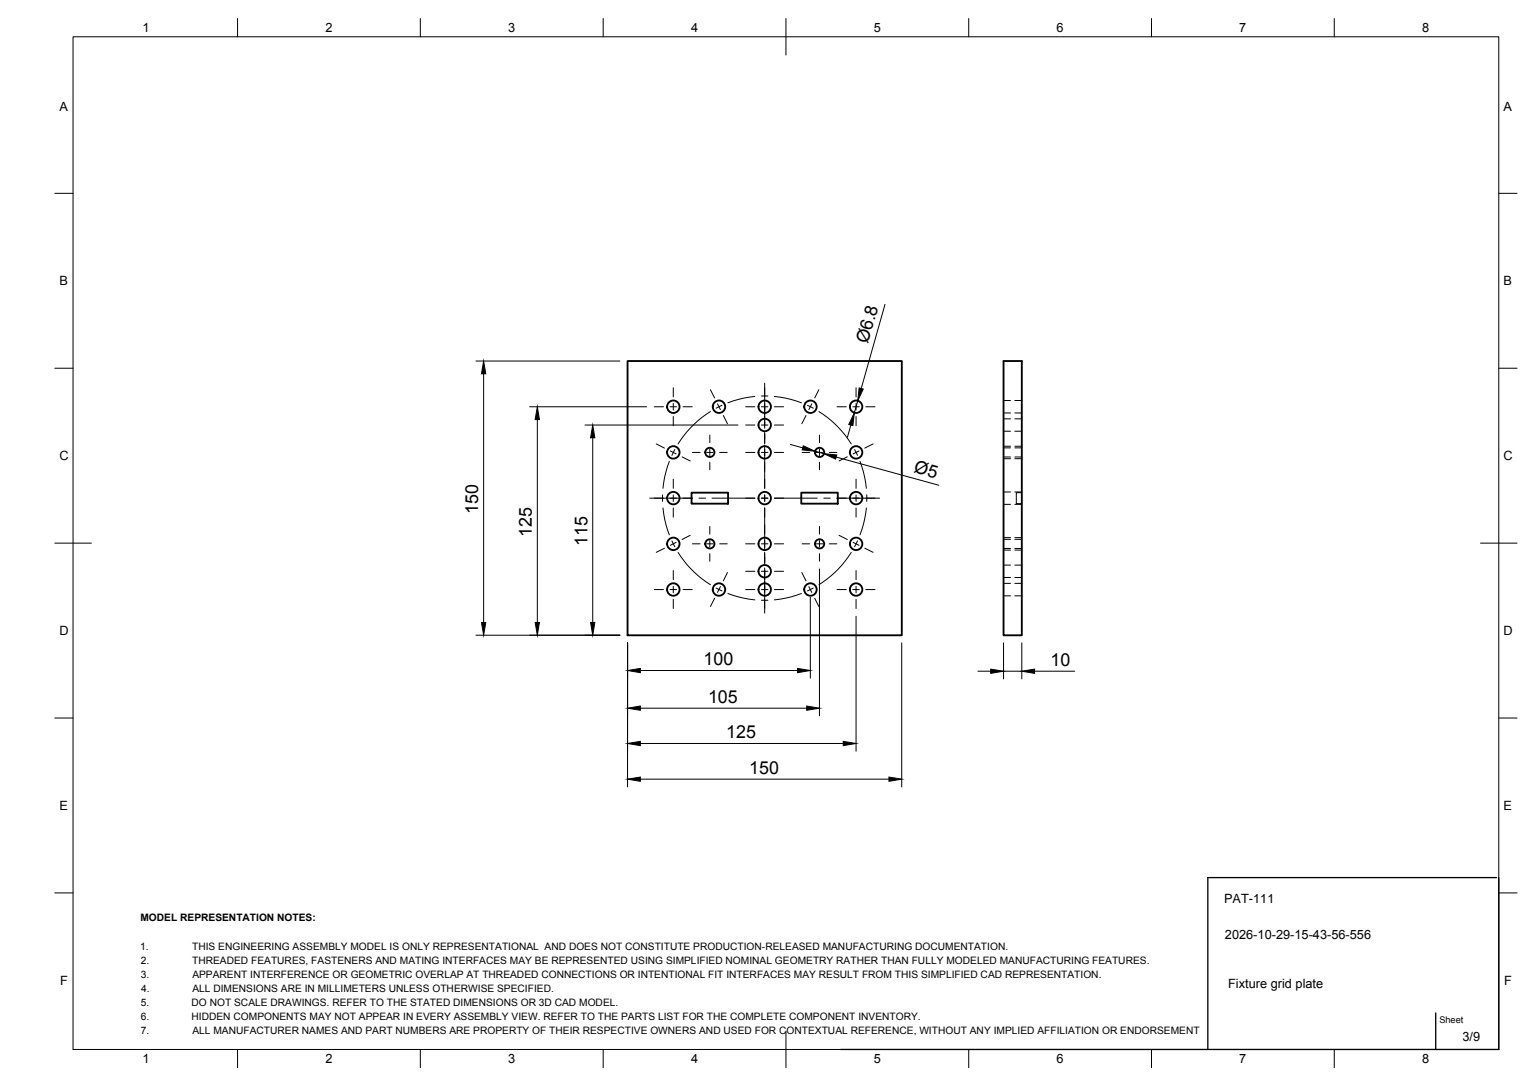
ISO-10303-21;
HEADER;
/* Generated by software containing ST-Developer
 * from STEP Tools, Inc. (www.steptools.com) 
 */

FILE_DESCRIPTION(
/* description */ ('Grid plate located blocks and clamp'),
/* implementation_level */ '2;1');

FILE_NAME(
/* name */ 'Fixture grid plate.step',
/* time_stamp */ '2026-10-29T15:43:47-07:00',
/* author */ (''),
/* organization */ (''),
/* preprocessor_version */ 'ST-DEVELOPER v20.2',
/* originating_system */ 'Autodesk Translation Framework v15.17.0.0',
/* authorisation */ '');

FILE_SCHEMA (('AUTOMOTIVE_DESIGN { 1 0 10303 214 3 1 1 }'));
ENDSEC;

DATA;
#10=MECHANICAL_DESIGN_GEOMETRIC_PRESENTATION_REPRESENTATION('',(#166),#5702);
#142=SHAPE_REPRESENTATION_RELATIONSHIP('SRR','None',#5760,#154);
#154=ADVANCED_BREP_SHAPE_REPRESENTATION('',(#180),#5690);
#166=STYLED_ITEM('',(#5911),#180);
#180=MANIFOLD_SOLID_BREP('Body1',#3261);
#192=FACE_BOUND('',#680,.T.);
#193=FACE_BOUND('',#681,.T.);
#194=FACE_BOUND('',#682,.T.);
#195=FACE_BOUND('',#683,.T.);
#196=FACE_BOUND('',#684,.T.);
#197=FACE_BOUND('',#685,.T.);
#198=FACE_BOUND('',#686,.T.);
#199=FACE_BOUND('',#687,.T.);
#200=FACE_BOUND('',#688,.T.);
#201=FACE_BOUND('',#689,.T.);
#202=FACE_BOUND('',#690,.T.);
#203=FACE_BOUND('',#691,.T.);
#204=FACE_BOUND('',#692,.T.);
#205=FACE_BOUND('',#693,.T.);
#206=FACE_BOUND('',#694,.T.);
#207=FACE_BOUND('',#695,.T.);
#208=FACE_BOUND('',#696,.T.);
#209=FACE_BOUND('',#697,.T.);
#210=FACE_BOUND('',#698,.T.);
#211=FACE_BOUND('',#699,.T.);
#212=FACE_BOUND('',#700,.T.);
#213=FACE_BOUND('',#701,.T.);
#214=FACE_BOUND('',#702,.T.);
#215=FACE_BOUND('',#703,.T.);
#216=FACE_BOUND('',#704,.T.);
#217=FACE_BOUND('',#705,.T.);
#218=FACE_BOUND('',#706,.T.);
#219=FACE_BOUND('',#708,.T.);
#220=FACE_BOUND('',#709,.T.);
#221=FACE_BOUND('',#710,.T.);
#222=FACE_BOUND('',#711,.T.);
#223=FACE_BOUND('',#712,.T.);
#224=FACE_BOUND('',#713,.T.);
#225=FACE_BOUND('',#714,.T.);
#226=FACE_BOUND('',#715,.T.);
#227=FACE_BOUND('',#716,.T.);
#228=FACE_BOUND('',#717,.T.);
#229=FACE_BOUND('',#718,.T.);
#230=FACE_BOUND('',#719,.T.);
#231=FACE_BOUND('',#720,.T.);
#232=FACE_BOUND('',#721,.T.);
#233=FACE_BOUND('',#722,.T.);
#234=FACE_BOUND('',#723,.T.);
#235=FACE_BOUND('',#724,.T.);
#236=FACE_BOUND('',#725,.T.);
#237=FACE_BOUND('',#726,.T.);
#238=FACE_BOUND('',#727,.T.);
#239=FACE_BOUND('',#728,.T.);
#240=FACE_BOUND('',#729,.T.);
#241=FACE_BOUND('',#730,.T.);
#242=FACE_BOUND('',#731,.T.);
#243=FACE_BOUND('',#732,.T.);
#268=CIRCLE('',#3423,0.25);
#269=CIRCLE('',#3424,0.25);
#270=CIRCLE('',#3426,0.25);
#271=CIRCLE('',#3427,0.25);
#272=CIRCLE('',#3429,0.25);
#273=CIRCLE('',#3430,0.25);
#274=CIRCLE('',#3432,0.25);
#275=CIRCLE('',#3433,0.25);
#276=CIRCLE('',#3435,0.34);
#277=CIRCLE('',#3436,0.34);
#278=CIRCLE('',#3438,0.34);
#279=CIRCLE('',#3439,0.34);
#280=CIRCLE('',#3441,0.34);
#281=CIRCLE('',#3442,0.34);
#282=CIRCLE('',#3444,0.34);
#283=CIRCLE('',#3445,0.34);
#284=CIRCLE('',#3447,0.34);
#285=CIRCLE('',#3448,0.34);
#286=CIRCLE('',#3450,0.34);
#287=CIRCLE('',#3451,0.34);
#288=CIRCLE('',#3453,0.34);
#289=CIRCLE('',#3454,0.34);
#290=CIRCLE('',#3456,0.34);
#291=CIRCLE('',#3457,0.34);
#292=CIRCLE('',#3459,0.34);
#293=CIRCLE('',#3460,0.34);
#294=CIRCLE('',#3462,0.34);
#295=CIRCLE('',#3463,0.34);
#296=CIRCLE('',#3465,0.34);
#297=CIRCLE('',#3466,0.34);
#298=CIRCLE('',#3468,0.34);
#299=CIRCLE('',#3469,0.34);
#300=CIRCLE('',#3471,0.34);
#301=CIRCLE('',#3472,0.34);
#302=CIRCLE('',#3474,0.34);
#303=CIRCLE('',#3475,0.34);
#304=CIRCLE('',#3477,0.34);
#305=CIRCLE('',#3478,0.34);
#306=CIRCLE('',#3480,0.34);
#307=CIRCLE('',#3481,0.34);
#308=CIRCLE('',#3483,0.34);
#309=CIRCLE('',#3484,0.34);
#310=CIRCLE('',#3486,0.34);
#311=CIRCLE('',#3487,0.34);
#312=CIRCLE('',#3489,0.34);
#313=CIRCLE('',#3490,0.34);
#314=CIRCLE('',#3492,0.34);
#315=CIRCLE('',#3493,0.34);
#316=CIRCLE('',#3495,0.34);
#317=CIRCLE('',#3496,0.34);
#397=CYLINDRICAL_SURFACE('',#3422,0.25);
#398=CYLINDRICAL_SURFACE('',#3425,0.25);
#399=CYLINDRICAL_SURFACE('',#3428,0.25);
#400=CYLINDRICAL_SURFACE('',#3431,0.25);
#401=CYLINDRICAL_SURFACE('',#3434,0.34);
#402=CYLINDRICAL_SURFACE('',#3437,0.34);
#403=CYLINDRICAL_SURFACE('',#3440,0.34);
#404=CYLINDRICAL_SURFACE('',#3443,0.34);
#405=CYLINDRICAL_SURFACE('',#3446,0.34);
#406=CYLINDRICAL_SURFACE('',#3449,0.34);
#407=CYLINDRICAL_SURFACE('',#3452,0.34);
#408=CYLINDRICAL_SURFACE('',#3455,0.34);
#409=CYLINDRICAL_SURFACE('',#3458,0.34);
#410=CYLINDRICAL_SURFACE('',#3461,0.34);
#411=CYLINDRICAL_SURFACE('',#3464,0.34);
#412=CYLINDRICAL_SURFACE('',#3467,0.34);
#413=CYLINDRICAL_SURFACE('',#3470,0.34);
#414=CYLINDRICAL_SURFACE('',#3473,0.34);
#415=CYLINDRICAL_SURFACE('',#3476,0.34);
#416=CYLINDRICAL_SURFACE('',#3479,0.34);
#417=CYLINDRICAL_SURFACE('',#3482,0.34);
#418=CYLINDRICAL_SURFACE('',#3485,0.34);
#419=CYLINDRICAL_SURFACE('',#3488,0.34);
#420=CYLINDRICAL_SURFACE('',#3491,0.34);
#421=CYLINDRICAL_SURFACE('',#3494,0.34);
#457=FACE_OUTER_BOUND('',#640,.T.);
#458=FACE_OUTER_BOUND('',#641,.T.);
#459=FACE_OUTER_BOUND('',#642,.T.);
#460=FACE_OUTER_BOUND('',#643,.T.);
#461=FACE_OUTER_BOUND('',#644,.T.);
#462=FACE_OUTER_BOUND('',#645,.T.);
#463=FACE_OUTER_BOUND('',#646,.T.);
#464=FACE_OUTER_BOUND('',#647,.T.);
#465=FACE_OUTER_BOUND('',#648,.T.);
#466=FACE_OUTER_BOUND('',#649,.T.);
#467=FACE_OUTER_BOUND('',#650,.T.);
#468=FACE_OUTER_BOUND('',#651,.T.);
#469=FACE_OUTER_BOUND('',#652,.T.);
#470=FACE_OUTER_BOUND('',#653,.T.);
#471=FACE_OUTER_BOUND('',#654,.T.);
#472=FACE_OUTER_BOUND('',#655,.T.);
#473=FACE_OUTER_BOUND('',#656,.T.);
#474=FACE_OUTER_BOUND('',#657,.T.);
#475=FACE_OUTER_BOUND('',#658,.T.);
#476=FACE_OUTER_BOUND('',#659,.T.);
#477=FACE_OUTER_BOUND('',#660,.T.);
#478=FACE_OUTER_BOUND('',#661,.T.);
#479=FACE_OUTER_BOUND('',#662,.T.);
#480=FACE_OUTER_BOUND('',#663,.T.);
#481=FACE_OUTER_BOUND('',#664,.T.);
#482=FACE_OUTER_BOUND('',#665,.T.);
#483=FACE_OUTER_BOUND('',#666,.T.);
#484=FACE_OUTER_BOUND('',#667,.T.);
#485=FACE_OUTER_BOUND('',#668,.T.);
#486=FACE_OUTER_BOUND('',#669,.T.);
#487=FACE_OUTER_BOUND('',#670,.T.);
#488=FACE_OUTER_BOUND('',#671,.T.);
#489=FACE_OUTER_BOUND('',#672,.T.);
#490=FACE_OUTER_BOUND('',#673,.T.);
#491=FACE_OUTER_BOUND('',#674,.T.);
#492=FACE_OUTER_BOUND('',#675,.T.);
#493=FACE_OUTER_BOUND('',#676,.T.);
#494=FACE_OUTER_BOUND('',#677,.T.);
#495=FACE_OUTER_BOUND('',#678,.T.);
#496=FACE_OUTER_BOUND('',#679,.T.);
#497=FACE_OUTER_BOUND('',#707,.T.);
#640=EDGE_LOOP('',(#2132,#2133,#2134,#2135));
#641=EDGE_LOOP('',(#2136,#2137,#2138,#2139));
#642=EDGE_LOOP('',(#2140,#2141,#2142,#2143));
#643=EDGE_LOOP('',(#2144,#2145,#2146,#2147));
#644=EDGE_LOOP('',(#2148,#2149,#2150,#2151));
#645=EDGE_LOOP('',(#2152,#2153,#2154,#2155));
#646=EDGE_LOOP('',(#2156,#2157,#2158,#2159));
#647=EDGE_LOOP('',(#2160,#2161,#2162,#2163));
#648=EDGE_LOOP('',(#2164,#2165,#2166,#2167));
#649=EDGE_LOOP('',(#2168,#2169,#2170,#2171));
#650=EDGE_LOOP('',(#2172,#2173,#2174,#2175));
#651=EDGE_LOOP('',(#2176,#2177,#2178,#2179));
#652=EDGE_LOOP('',(#2180,#2181,#2182,#2183));
#653=EDGE_LOOP('',(#2184,#2185,#2186,#2187));
#654=EDGE_LOOP('',(#2188,#2189,#2190,#2191));
#655=EDGE_LOOP('',(#2192,#2193,#2194,#2195));
#656=EDGE_LOOP('',(#2196,#2197,#2198,#2199));
#657=EDGE_LOOP('',(#2200,#2201,#2202,#2203));
#658=EDGE_LOOP('',(#2204,#2205,#2206,#2207));
#659=EDGE_LOOP('',(#2208,#2209,#2210,#2211));
#660=EDGE_LOOP('',(#2212,#2213,#2214,#2215));
#661=EDGE_LOOP('',(#2216,#2217,#2218,#2219));
#662=EDGE_LOOP('',(#2220,#2221,#2222,#2223));
#663=EDGE_LOOP('',(#2224,#2225,#2226,#2227));
#664=EDGE_LOOP('',(#2228,#2229,#2230,#2231));
#665=EDGE_LOOP('',(#2232,#2233,#2234,#2235));
#666=EDGE_LOOP('',(#2236,#2237,#2238,#2239));
#667=EDGE_LOOP('',(#2240,#2241,#2242,#2243));
#668=EDGE_LOOP('',(#2244,#2245,#2246,#2247));
#669=EDGE_LOOP('',(#2248,#2249,#2250,#2251));
#670=EDGE_LOOP('',(#2252,#2253,#2254,#2255));
#671=EDGE_LOOP('',(#2256,#2257,#2258,#2259));
#672=EDGE_LOOP('',(#2260,#2261,#2262,#2263));
#673=EDGE_LOOP('',(#2264,#2265,#2266,#2267));
#674=EDGE_LOOP('',(#2268,#2269,#2270,#2271));
#675=EDGE_LOOP('',(#2272,#2273,#2274,#2275));
#676=EDGE_LOOP('',(#2276,#2277,#2278,#2279));
#677=EDGE_LOOP('',(#2280,#2281,#2282,#2283));
#678=EDGE_LOOP('',(#2284,#2285,#2286,#2287));
#679=EDGE_LOOP('',(#2288,#2289,#2290,#2291));
#680=EDGE_LOOP('',(#2292,#2293,#2294,#2295));
#681=EDGE_LOOP('',(#2296));
#682=EDGE_LOOP('',(#2297));
#683=EDGE_LOOP('',(#2298));
#684=EDGE_LOOP('',(#2299));
#685=EDGE_LOOP('',(#2300));
#686=EDGE_LOOP('',(#2301));
#687=EDGE_LOOP('',(#2302));
#688=EDGE_LOOP('',(#2303));
#689=EDGE_LOOP('',(#2304));
#690=EDGE_LOOP('',(#2305));
#691=EDGE_LOOP('',(#2306));
#692=EDGE_LOOP('',(#2307));
#693=EDGE_LOOP('',(#2308));
#694=EDGE_LOOP('',(#2309));
#695=EDGE_LOOP('',(#2310));
#696=EDGE_LOOP('',(#2311));
#697=EDGE_LOOP('',(#2312));
#698=EDGE_LOOP('',(#2313));
#699=EDGE_LOOP('',(#2314));
#700=EDGE_LOOP('',(#2315));
#701=EDGE_LOOP('',(#2316));
#702=EDGE_LOOP('',(#2317));
#703=EDGE_LOOP('',(#2318));
#704=EDGE_LOOP('',(#2319));
#705=EDGE_LOOP('',(#2320));
#706=EDGE_LOOP('',(#2321,#2322,#2323,#2324));
#707=EDGE_LOOP('',(#2325,#2326,#2327,#2328));
#708=EDGE_LOOP('',(#2329));
#709=EDGE_LOOP('',(#2330));
#710=EDGE_LOOP('',(#2331));
#711=EDGE_LOOP('',(#2332));
#712=EDGE_LOOP('',(#2333));
#713=EDGE_LOOP('',(#2334));
#714=EDGE_LOOP('',(#2335));
#715=EDGE_LOOP('',(#2336));
#716=EDGE_LOOP('',(#2337));
#717=EDGE_LOOP('',(#2338));
#718=EDGE_LOOP('',(#2339));
#719=EDGE_LOOP('',(#2340));
#720=EDGE_LOOP('',(#2341));
#721=EDGE_LOOP('',(#2342));
#722=EDGE_LOOP('',(#2343));
#723=EDGE_LOOP('',(#2344));
#724=EDGE_LOOP('',(#2345));
#725=EDGE_LOOP('',(#2346));
#726=EDGE_LOOP('',(#2347));
#727=EDGE_LOOP('',(#2348));
#728=EDGE_LOOP('',(#2349));
#729=EDGE_LOOP('',(#2350));
#730=EDGE_LOOP('',(#2351));
#731=EDGE_LOOP('',(#2352));
#732=EDGE_LOOP('',(#2353));
#899=LINE('',#4747,#1172);
#900=LINE('',#4749,#1173);
#901=LINE('',#4751,#1174);
#902=LINE('',#4752,#1175);
#903=LINE('',#4755,#1176);
#904=LINE('',#4757,#1177);
#905=LINE('',#4758,#1178);
#906=LINE('',#4761,#1179);
#907=LINE('',#4763,#1180);
#908=LINE('',#4764,#1181);
#909=LINE('',#4766,#1182);
#910=LINE('',#4767,#1183);
#911=LINE('',#4772,#1184);
#912=LINE('',#4774,#1185);
#913=LINE('',#4776,#1186);
#914=LINE('',#4777,#1187);
#915=LINE('',#4780,#1188);
#916=LINE('',#4782,#1189);
#917=LINE('',#4783,#1190);
#918=LINE('',#4786,#1191);
#919=LINE('',#4788,#1192);
#920=LINE('',#4789,#1193);
#921=LINE('',#4791,#1194);
#922=LINE('',#4792,#1195);
#923=LINE('',#4798,#1196);
#924=LINE('',#4804,#1197);
#925=LINE('',#4810,#1198);
#926=LINE('',#4816,#1199);
#927=LINE('',#4822,#1200);
#928=LINE('',#4828,#1201);
#929=LINE('',#4834,#1202);
#930=LINE('',#4840,#1203);
#931=LINE('',#4846,#1204);
#932=LINE('',#4852,#1205);
#933=LINE('',#4858,#1206);
#934=LINE('',#4864,#1207);
#935=LINE('',#4870,#1208);
#936=LINE('',#4876,#1209);
#937=LINE('',#4882,#1210);
#938=LINE('',#4888,#1211);
#939=LINE('',#4894,#1212);
#940=LINE('',#4900,#1213);
#941=LINE('',#4906,#1214);
#942=LINE('',#4912,#1215);
#943=LINE('',#4918,#1216);
#944=LINE('',#4924,#1217);
#945=LINE('',#4930,#1218);
#946=LINE('',#4936,#1219);
#947=LINE('',#4942,#1220);
#948=LINE('',#4947,#1221);
#949=LINE('',#4949,#1222);
#950=LINE('',#4951,#1223);
#951=LINE('',#4952,#1224);
#952=LINE('',#4955,#1225);
#953=LINE('',#4957,#1226);
#954=LINE('',#4958,#1227);
#955=LINE('',#4961,#1228);
#956=LINE('',#4963,#1229);
#957=LINE('',#4964,#1230);
#958=LINE('',#4966,#1231);
#959=LINE('',#4967,#1232);
#1172=VECTOR('',#3769,1.);
#1173=VECTOR('',#3770,1.);
#1174=VECTOR('',#3771,1.);
#1175=VECTOR('',#3772,1.);
#1176=VECTOR('',#3775,1.);
#1177=VECTOR('',#3776,1.);
#1178=VECTOR('',#3777,1.);
#1179=VECTOR('',#3780,1.);
#1180=VECTOR('',#3781,1.);
#1181=VECTOR('',#3782,1.);
#1182=VECTOR('',#3785,1.);
#1183=VECTOR('',#3786,1.);
#1184=VECTOR('',#3791,1.);
#1185=VECTOR('',#3792,1.);
#1186=VECTOR('',#3793,1.);
#1187=VECTOR('',#3794,1.);
#1188=VECTOR('',#3797,1.);
#1189=VECTOR('',#3798,1.);
#1190=VECTOR('',#3799,1.);
#1191=VECTOR('',#3802,1.);
#1192=VECTOR('',#3803,1.);
#1193=VECTOR('',#3804,1.);
#1194=VECTOR('',#3807,1.);
#1195=VECTOR('',#3808,1.);
#1196=VECTOR('',#3815,0.25);
#1197=VECTOR('',#3822,0.25);
#1198=VECTOR('',#3829,0.25);
#1199=VECTOR('',#3836,0.25);
#1200=VECTOR('',#3843,0.34);
#1201=VECTOR('',#3850,0.34);
#1202=VECTOR('',#3857,0.34);
#1203=VECTOR('',#3864,0.34);
#1204=VECTOR('',#3871,0.34);
#1205=VECTOR('',#3878,0.34);
#1206=VECTOR('',#3885,0.34);
#1207=VECTOR('',#3892,0.34);
#1208=VECTOR('',#3899,0.34);
#1209=VECTOR('',#3906,0.34);
#1210=VECTOR('',#3913,0.34);
#1211=VECTOR('',#3920,0.34);
#1212=VECTOR('',#3927,0.34);
#1213=VECTOR('',#3934,0.34);
#1214=VECTOR('',#3941,0.34);
#1215=VECTOR('',#3948,0.34);
#1216=VECTOR('',#3955,0.34);
#1217=VECTOR('',#3962,0.34);
#1218=VECTOR('',#3969,0.34);
#1219=VECTOR('',#3976,0.34);
#1220=VECTOR('',#3983,0.34);
#1221=VECTOR('',#3988,1.);
#1222=VECTOR('',#3989,1.);
#1223=VECTOR('',#3990,1.);
#1224=VECTOR('',#3991,1.);
#1225=VECTOR('',#3994,1.);
#1226=VECTOR('',#3995,1.);
#1227=VECTOR('',#3996,1.);
#1228=VECTOR('',#3999,1.);
#1229=VECTOR('',#4000,1.);
#1230=VECTOR('',#4001,1.);
#1231=VECTOR('',#4004,1.);
#1232=VECTOR('',#4005,1.);
#1445=VERTEX_POINT('',#4745);
#1446=VERTEX_POINT('',#4746);
#1447=VERTEX_POINT('',#4748);
#1448=VERTEX_POINT('',#4750);
#1449=VERTEX_POINT('',#4754);
#1450=VERTEX_POINT('',#4756);
#1451=VERTEX_POINT('',#4760);
#1452=VERTEX_POINT('',#4762);
#1453=VERTEX_POINT('',#4770);
#1454=VERTEX_POINT('',#4771);
#1455=VERTEX_POINT('',#4773);
#1456=VERTEX_POINT('',#4775);
#1457=VERTEX_POINT('',#4779);
#1458=VERTEX_POINT('',#4781);
#1459=VERTEX_POINT('',#4785);
#1460=VERTEX_POINT('',#4787);
#1461=VERTEX_POINT('',#4795);
#1462=VERTEX_POINT('',#4797);
#1463=VERTEX_POINT('',#4801);
#1464=VERTEX_POINT('',#4803);
#1465=VERTEX_POINT('',#4807);
#1466=VERTEX_POINT('',#4809);
#1467=VERTEX_POINT('',#4813);
#1468=VERTEX_POINT('',#4815);
#1469=VERTEX_POINT('',#4819);
#1470=VERTEX_POINT('',#4821);
#1471=VERTEX_POINT('',#4825);
#1472=VERTEX_POINT('',#4827);
#1473=VERTEX_POINT('',#4831);
#1474=VERTEX_POINT('',#4833);
#1475=VERTEX_POINT('',#4837);
#1476=VERTEX_POINT('',#4839);
#1477=VERTEX_POINT('',#4843);
#1478=VERTEX_POINT('',#4845);
#1479=VERTEX_POINT('',#4849);
#1480=VERTEX_POINT('',#4851);
#1481=VERTEX_POINT('',#4855);
#1482=VERTEX_POINT('',#4857);
#1483=VERTEX_POINT('',#4861);
#1484=VERTEX_POINT('',#4863);
#1485=VERTEX_POINT('',#4867);
#1486=VERTEX_POINT('',#4869);
#1487=VERTEX_POINT('',#4873);
#1488=VERTEX_POINT('',#4875);
#1489=VERTEX_POINT('',#4879);
#1490=VERTEX_POINT('',#4881);
#1491=VERTEX_POINT('',#4885);
#1492=VERTEX_POINT('',#4887);
#1493=VERTEX_POINT('',#4891);
#1494=VERTEX_POINT('',#4893);
#1495=VERTEX_POINT('',#4897);
#1496=VERTEX_POINT('',#4899);
#1497=VERTEX_POINT('',#4903);
#1498=VERTEX_POINT('',#4905);
#1499=VERTEX_POINT('',#4909);
#1500=VERTEX_POINT('',#4911);
#1501=VERTEX_POINT('',#4915);
#1502=VERTEX_POINT('',#4917);
#1503=VERTEX_POINT('',#4921);
#1504=VERTEX_POINT('',#4923);
#1505=VERTEX_POINT('',#4927);
#1506=VERTEX_POINT('',#4929);
#1507=VERTEX_POINT('',#4933);
#1508=VERTEX_POINT('',#4935);
#1509=VERTEX_POINT('',#4939);
#1510=VERTEX_POINT('',#4941);
#1511=VERTEX_POINT('',#4945);
#1512=VERTEX_POINT('',#4946);
#1513=VERTEX_POINT('',#4948);
#1514=VERTEX_POINT('',#4950);
#1515=VERTEX_POINT('',#4954);
#1516=VERTEX_POINT('',#4956);
#1517=VERTEX_POINT('',#4960);
#1518=VERTEX_POINT('',#4962);
#1716=EDGE_CURVE('',#1445,#1446,#899,.T.);
#1717=EDGE_CURVE('',#1447,#1445,#900,.T.);
#1718=EDGE_CURVE('',#1448,#1447,#901,.T.);
#1719=EDGE_CURVE('',#1448,#1446,#902,.T.);
#1720=EDGE_CURVE('',#1446,#1449,#903,.T.);
#1721=EDGE_CURVE('',#1450,#1448,#904,.T.);
#1722=EDGE_CURVE('',#1450,#1449,#905,.T.);
#1723=EDGE_CURVE('',#1449,#1451,#906,.T.);
#1724=EDGE_CURVE('',#1452,#1450,#907,.T.);
#1725=EDGE_CURVE('',#1452,#1451,#908,.T.);
#1726=EDGE_CURVE('',#1451,#1445,#909,.T.);
#1727=EDGE_CURVE('',#1447,#1452,#910,.T.);
#1728=EDGE_CURVE('',#1453,#1454,#911,.T.);
#1729=EDGE_CURVE('',#1455,#1453,#912,.T.);
#1730=EDGE_CURVE('',#1456,#1455,#913,.T.);
#1731=EDGE_CURVE('',#1456,#1454,#914,.T.);
#1732=EDGE_CURVE('',#1454,#1457,#915,.T.);
#1733=EDGE_CURVE('',#1458,#1456,#916,.T.);
#1734=EDGE_CURVE('',#1458,#1457,#917,.T.);
#1735=EDGE_CURVE('',#1457,#1459,#918,.T.);
#1736=EDGE_CURVE('',#1460,#1458,#919,.T.);
#1737=EDGE_CURVE('',#1460,#1459,#920,.T.);
#1738=EDGE_CURVE('',#1459,#1453,#921,.T.);
#1739=EDGE_CURVE('',#1455,#1460,#922,.T.);
#1740=EDGE_CURVE('',#1461,#1461,#268,.T.);
#1741=EDGE_CURVE('',#1461,#1462,#923,.T.);
#1742=EDGE_CURVE('',#1462,#1462,#269,.T.);
#1743=EDGE_CURVE('',#1463,#1463,#270,.T.);
#1744=EDGE_CURVE('',#1463,#1464,#924,.T.);
#1745=EDGE_CURVE('',#1464,#1464,#271,.T.);
#1746=EDGE_CURVE('',#1465,#1465,#272,.T.);
#1747=EDGE_CURVE('',#1465,#1466,#925,.T.);
#1748=EDGE_CURVE('',#1466,#1466,#273,.T.);
#1749=EDGE_CURVE('',#1467,#1467,#274,.T.);
#1750=EDGE_CURVE('',#1467,#1468,#926,.T.);
#1751=EDGE_CURVE('',#1468,#1468,#275,.T.);
#1752=EDGE_CURVE('',#1469,#1469,#276,.T.);
#1753=EDGE_CURVE('',#1469,#1470,#927,.T.);
#1754=EDGE_CURVE('',#1470,#1470,#277,.T.);
#1755=EDGE_CURVE('',#1471,#1471,#278,.T.);
#1756=EDGE_CURVE('',#1471,#1472,#928,.T.);
#1757=EDGE_CURVE('',#1472,#1472,#279,.T.);
#1758=EDGE_CURVE('',#1473,#1473,#280,.T.);
#1759=EDGE_CURVE('',#1473,#1474,#929,.T.);
#1760=EDGE_CURVE('',#1474,#1474,#281,.T.);
#1761=EDGE_CURVE('',#1475,#1475,#282,.T.);
#1762=EDGE_CURVE('',#1475,#1476,#930,.T.);
#1763=EDGE_CURVE('',#1476,#1476,#283,.T.);
#1764=EDGE_CURVE('',#1477,#1477,#284,.T.);
#1765=EDGE_CURVE('',#1477,#1478,#931,.T.);
#1766=EDGE_CURVE('',#1478,#1478,#285,.T.);
#1767=EDGE_CURVE('',#1479,#1479,#286,.T.);
#1768=EDGE_CURVE('',#1479,#1480,#932,.T.);
#1769=EDGE_CURVE('',#1480,#1480,#287,.T.);
#1770=EDGE_CURVE('',#1481,#1481,#288,.T.);
#1771=EDGE_CURVE('',#1481,#1482,#933,.T.);
#1772=EDGE_CURVE('',#1482,#1482,#289,.T.);
#1773=EDGE_CURVE('',#1483,#1483,#290,.T.);
#1774=EDGE_CURVE('',#1483,#1484,#934,.T.);
#1775=EDGE_CURVE('',#1484,#1484,#291,.T.);
#1776=EDGE_CURVE('',#1485,#1485,#292,.T.);
#1777=EDGE_CURVE('',#1485,#1486,#935,.T.);
#1778=EDGE_CURVE('',#1486,#1486,#293,.T.);
#1779=EDGE_CURVE('',#1487,#1487,#294,.T.);
#1780=EDGE_CURVE('',#1487,#1488,#936,.T.);
#1781=EDGE_CURVE('',#1488,#1488,#295,.T.);
#1782=EDGE_CURVE('',#1489,#1489,#296,.T.);
#1783=EDGE_CURVE('',#1489,#1490,#937,.T.);
#1784=EDGE_CURVE('',#1490,#1490,#297,.T.);
#1785=EDGE_CURVE('',#1491,#1491,#298,.T.);
#1786=EDGE_CURVE('',#1491,#1492,#938,.T.);
#1787=EDGE_CURVE('',#1492,#1492,#299,.T.);
#1788=EDGE_CURVE('',#1493,#1493,#300,.T.);
#1789=EDGE_CURVE('',#1493,#1494,#939,.T.);
#1790=EDGE_CURVE('',#1494,#1494,#301,.T.);
#1791=EDGE_CURVE('',#1495,#1495,#302,.T.);
#1792=EDGE_CURVE('',#1495,#1496,#940,.T.);
#1793=EDGE_CURVE('',#1496,#1496,#303,.T.);
#1794=EDGE_CURVE('',#1497,#1497,#304,.T.);
#1795=EDGE_CURVE('',#1497,#1498,#941,.T.);
#1796=EDGE_CURVE('',#1498,#1498,#305,.T.);
#1797=EDGE_CURVE('',#1499,#1499,#306,.T.);
#1798=EDGE_CURVE('',#1499,#1500,#942,.T.);
#1799=EDGE_CURVE('',#1500,#1500,#307,.T.);
#1800=EDGE_CURVE('',#1501,#1501,#308,.T.);
#1801=EDGE_CURVE('',#1501,#1502,#943,.T.);
#1802=EDGE_CURVE('',#1502,#1502,#309,.T.);
#1803=EDGE_CURVE('',#1503,#1503,#310,.T.);
#1804=EDGE_CURVE('',#1503,#1504,#944,.T.);
#1805=EDGE_CURVE('',#1504,#1504,#311,.T.);
#1806=EDGE_CURVE('',#1505,#1505,#312,.T.);
#1807=EDGE_CURVE('',#1505,#1506,#945,.T.);
#1808=EDGE_CURVE('',#1506,#1506,#313,.T.);
#1809=EDGE_CURVE('',#1507,#1507,#314,.T.);
#1810=EDGE_CURVE('',#1507,#1508,#946,.T.);
#1811=EDGE_CURVE('',#1508,#1508,#315,.T.);
#1812=EDGE_CURVE('',#1509,#1509,#316,.T.);
#1813=EDGE_CURVE('',#1509,#1510,#947,.T.);
#1814=EDGE_CURVE('',#1510,#1510,#317,.T.);
#1815=EDGE_CURVE('',#1511,#1512,#948,.T.);
#1816=EDGE_CURVE('',#1512,#1513,#949,.T.);
#1817=EDGE_CURVE('',#1514,#1513,#950,.T.);
#1818=EDGE_CURVE('',#1511,#1514,#951,.T.);
#1819=EDGE_CURVE('',#1515,#1511,#952,.T.);
#1820=EDGE_CURVE('',#1516,#1514,#953,.T.);
#1821=EDGE_CURVE('',#1515,#1516,#954,.T.);
#1822=EDGE_CURVE('',#1517,#1515,#955,.T.);
#1823=EDGE_CURVE('',#1518,#1516,#956,.T.);
#1824=EDGE_CURVE('',#1517,#1518,#957,.T.);
#1825=EDGE_CURVE('',#1512,#1517,#958,.T.);
#1826=EDGE_CURVE('',#1513,#1518,#959,.T.);
#2132=ORIENTED_EDGE('',*,*,#1716,.F.);
#2133=ORIENTED_EDGE('',*,*,#1717,.F.);
#2134=ORIENTED_EDGE('',*,*,#1718,.F.);
#2135=ORIENTED_EDGE('',*,*,#1719,.T.);
#2136=ORIENTED_EDGE('',*,*,#1720,.F.);
#2137=ORIENTED_EDGE('',*,*,#1719,.F.);
#2138=ORIENTED_EDGE('',*,*,#1721,.F.);
#2139=ORIENTED_EDGE('',*,*,#1722,.T.);
#2140=ORIENTED_EDGE('',*,*,#1723,.F.);
#2141=ORIENTED_EDGE('',*,*,#1722,.F.);
#2142=ORIENTED_EDGE('',*,*,#1724,.F.);
#2143=ORIENTED_EDGE('',*,*,#1725,.T.);
#2144=ORIENTED_EDGE('',*,*,#1726,.F.);
#2145=ORIENTED_EDGE('',*,*,#1725,.F.);
#2146=ORIENTED_EDGE('',*,*,#1727,.F.);
#2147=ORIENTED_EDGE('',*,*,#1717,.T.);
#2148=ORIENTED_EDGE('',*,*,#1721,.T.);
#2149=ORIENTED_EDGE('',*,*,#1718,.T.);
#2150=ORIENTED_EDGE('',*,*,#1727,.T.);
#2151=ORIENTED_EDGE('',*,*,#1724,.T.);
#2152=ORIENTED_EDGE('',*,*,#1728,.F.);
#2153=ORIENTED_EDGE('',*,*,#1729,.F.);
#2154=ORIENTED_EDGE('',*,*,#1730,.F.);
#2155=ORIENTED_EDGE('',*,*,#1731,.T.);
#2156=ORIENTED_EDGE('',*,*,#1732,.F.);
#2157=ORIENTED_EDGE('',*,*,#1731,.F.);
#2158=ORIENTED_EDGE('',*,*,#1733,.F.);
#2159=ORIENTED_EDGE('',*,*,#1734,.T.);
#2160=ORIENTED_EDGE('',*,*,#1735,.F.);
#2161=ORIENTED_EDGE('',*,*,#1734,.F.);
#2162=ORIENTED_EDGE('',*,*,#1736,.F.);
#2163=ORIENTED_EDGE('',*,*,#1737,.T.);
#2164=ORIENTED_EDGE('',*,*,#1738,.F.);
#2165=ORIENTED_EDGE('',*,*,#1737,.F.);
#2166=ORIENTED_EDGE('',*,*,#1739,.F.);
#2167=ORIENTED_EDGE('',*,*,#1729,.T.);
#2168=ORIENTED_EDGE('',*,*,#1733,.T.);
#2169=ORIENTED_EDGE('',*,*,#1730,.T.);
#2170=ORIENTED_EDGE('',*,*,#1739,.T.);
#2171=ORIENTED_EDGE('',*,*,#1736,.T.);
#2172=ORIENTED_EDGE('',*,*,#1740,.F.);
#2173=ORIENTED_EDGE('',*,*,#1741,.T.);
#2174=ORIENTED_EDGE('',*,*,#1742,.F.);
#2175=ORIENTED_EDGE('',*,*,#1741,.F.);
#2176=ORIENTED_EDGE('',*,*,#1743,.F.);
#2177=ORIENTED_EDGE('',*,*,#1744,.T.);
#2178=ORIENTED_EDGE('',*,*,#1745,.F.);
#2179=ORIENTED_EDGE('',*,*,#1744,.F.);
#2180=ORIENTED_EDGE('',*,*,#1746,.F.);
#2181=ORIENTED_EDGE('',*,*,#1747,.T.);
#2182=ORIENTED_EDGE('',*,*,#1748,.F.);
#2183=ORIENTED_EDGE('',*,*,#1747,.F.);
#2184=ORIENTED_EDGE('',*,*,#1749,.F.);
#2185=ORIENTED_EDGE('',*,*,#1750,.T.);
#2186=ORIENTED_EDGE('',*,*,#1751,.F.);
#2187=ORIENTED_EDGE('',*,*,#1750,.F.);
#2188=ORIENTED_EDGE('',*,*,#1752,.F.);
#2189=ORIENTED_EDGE('',*,*,#1753,.T.);
#2190=ORIENTED_EDGE('',*,*,#1754,.F.);
#2191=ORIENTED_EDGE('',*,*,#1753,.F.);
#2192=ORIENTED_EDGE('',*,*,#1755,.F.);
#2193=ORIENTED_EDGE('',*,*,#1756,.T.);
#2194=ORIENTED_EDGE('',*,*,#1757,.F.);
#2195=ORIENTED_EDGE('',*,*,#1756,.F.);
#2196=ORIENTED_EDGE('',*,*,#1758,.F.);
#2197=ORIENTED_EDGE('',*,*,#1759,.T.);
#2198=ORIENTED_EDGE('',*,*,#1760,.F.);
#2199=ORIENTED_EDGE('',*,*,#1759,.F.);
#2200=ORIENTED_EDGE('',*,*,#1761,.F.);
#2201=ORIENTED_EDGE('',*,*,#1762,.T.);
#2202=ORIENTED_EDGE('',*,*,#1763,.F.);
#2203=ORIENTED_EDGE('',*,*,#1762,.F.);
#2204=ORIENTED_EDGE('',*,*,#1764,.F.);
#2205=ORIENTED_EDGE('',*,*,#1765,.T.);
#2206=ORIENTED_EDGE('',*,*,#1766,.F.);
#2207=ORIENTED_EDGE('',*,*,#1765,.F.);
#2208=ORIENTED_EDGE('',*,*,#1767,.F.);
#2209=ORIENTED_EDGE('',*,*,#1768,.T.);
#2210=ORIENTED_EDGE('',*,*,#1769,.F.);
#2211=ORIENTED_EDGE('',*,*,#1768,.F.);
#2212=ORIENTED_EDGE('',*,*,#1770,.F.);
#2213=ORIENTED_EDGE('',*,*,#1771,.T.);
#2214=ORIENTED_EDGE('',*,*,#1772,.F.);
#2215=ORIENTED_EDGE('',*,*,#1771,.F.);
#2216=ORIENTED_EDGE('',*,*,#1773,.F.);
#2217=ORIENTED_EDGE('',*,*,#1774,.T.);
#2218=ORIENTED_EDGE('',*,*,#1775,.F.);
#2219=ORIENTED_EDGE('',*,*,#1774,.F.);
#2220=ORIENTED_EDGE('',*,*,#1776,.F.);
#2221=ORIENTED_EDGE('',*,*,#1777,.T.);
#2222=ORIENTED_EDGE('',*,*,#1778,.F.);
#2223=ORIENTED_EDGE('',*,*,#1777,.F.);
#2224=ORIENTED_EDGE('',*,*,#1779,.F.);
#2225=ORIENTED_EDGE('',*,*,#1780,.T.);
#2226=ORIENTED_EDGE('',*,*,#1781,.F.);
#2227=ORIENTED_EDGE('',*,*,#1780,.F.);
#2228=ORIENTED_EDGE('',*,*,#1782,.F.);
#2229=ORIENTED_EDGE('',*,*,#1783,.T.);
#2230=ORIENTED_EDGE('',*,*,#1784,.F.);
#2231=ORIENTED_EDGE('',*,*,#1783,.F.);
#2232=ORIENTED_EDGE('',*,*,#1785,.F.);
#2233=ORIENTED_EDGE('',*,*,#1786,.T.);
#2234=ORIENTED_EDGE('',*,*,#1787,.F.);
#2235=ORIENTED_EDGE('',*,*,#1786,.F.);
#2236=ORIENTED_EDGE('',*,*,#1788,.F.);
#2237=ORIENTED_EDGE('',*,*,#1789,.T.);
#2238=ORIENTED_EDGE('',*,*,#1790,.F.);
#2239=ORIENTED_EDGE('',*,*,#1789,.F.);
#2240=ORIENTED_EDGE('',*,*,#1791,.F.);
#2241=ORIENTED_EDGE('',*,*,#1792,.T.);
#2242=ORIENTED_EDGE('',*,*,#1793,.F.);
#2243=ORIENTED_EDGE('',*,*,#1792,.F.);
#2244=ORIENTED_EDGE('',*,*,#1794,.F.);
#2245=ORIENTED_EDGE('',*,*,#1795,.T.);
#2246=ORIENTED_EDGE('',*,*,#1796,.F.);
#2247=ORIENTED_EDGE('',*,*,#1795,.F.);
#2248=ORIENTED_EDGE('',*,*,#1797,.F.);
#2249=ORIENTED_EDGE('',*,*,#1798,.T.);
#2250=ORIENTED_EDGE('',*,*,#1799,.F.);
#2251=ORIENTED_EDGE('',*,*,#1798,.F.);
#2252=ORIENTED_EDGE('',*,*,#1800,.F.);
#2253=ORIENTED_EDGE('',*,*,#1801,.T.);
#2254=ORIENTED_EDGE('',*,*,#1802,.F.);
#2255=ORIENTED_EDGE('',*,*,#1801,.F.);
#2256=ORIENTED_EDGE('',*,*,#1803,.F.);
#2257=ORIENTED_EDGE('',*,*,#1804,.T.);
#2258=ORIENTED_EDGE('',*,*,#1805,.F.);
#2259=ORIENTED_EDGE('',*,*,#1804,.F.);
#2260=ORIENTED_EDGE('',*,*,#1806,.F.);
#2261=ORIENTED_EDGE('',*,*,#1807,.T.);
#2262=ORIENTED_EDGE('',*,*,#1808,.F.);
#2263=ORIENTED_EDGE('',*,*,#1807,.F.);
#2264=ORIENTED_EDGE('',*,*,#1809,.F.);
#2265=ORIENTED_EDGE('',*,*,#1810,.T.);
#2266=ORIENTED_EDGE('',*,*,#1811,.F.);
#2267=ORIENTED_EDGE('',*,*,#1810,.F.);
#2268=ORIENTED_EDGE('',*,*,#1812,.F.);
#2269=ORIENTED_EDGE('',*,*,#1813,.T.);
#2270=ORIENTED_EDGE('',*,*,#1814,.F.);
#2271=ORIENTED_EDGE('',*,*,#1813,.F.);
#2272=ORIENTED_EDGE('',*,*,#1815,.T.);
#2273=ORIENTED_EDGE('',*,*,#1816,.T.);
#2274=ORIENTED_EDGE('',*,*,#1817,.F.);
#2275=ORIENTED_EDGE('',*,*,#1818,.F.);
#2276=ORIENTED_EDGE('',*,*,#1819,.T.);
#2277=ORIENTED_EDGE('',*,*,#1818,.T.);
#2278=ORIENTED_EDGE('',*,*,#1820,.F.);
#2279=ORIENTED_EDGE('',*,*,#1821,.F.);
#2280=ORIENTED_EDGE('',*,*,#1822,.T.);
#2281=ORIENTED_EDGE('',*,*,#1821,.T.);
#2282=ORIENTED_EDGE('',*,*,#1823,.F.);
#2283=ORIENTED_EDGE('',*,*,#1824,.F.);
#2284=ORIENTED_EDGE('',*,*,#1825,.T.);
#2285=ORIENTED_EDGE('',*,*,#1824,.T.);
#2286=ORIENTED_EDGE('',*,*,#1826,.F.);
#2287=ORIENTED_EDGE('',*,*,#1816,.F.);
#2288=ORIENTED_EDGE('',*,*,#1826,.T.);
#2289=ORIENTED_EDGE('',*,*,#1823,.T.);
#2290=ORIENTED_EDGE('',*,*,#1820,.T.);
#2291=ORIENTED_EDGE('',*,*,#1817,.T.);
#2292=ORIENTED_EDGE('',*,*,#1735,.T.);
#2293=ORIENTED_EDGE('',*,*,#1738,.T.);
#2294=ORIENTED_EDGE('',*,*,#1728,.T.);
#2295=ORIENTED_EDGE('',*,*,#1732,.T.);
#2296=ORIENTED_EDGE('',*,*,#1754,.T.);
#2297=ORIENTED_EDGE('',*,*,#1757,.T.);
#2298=ORIENTED_EDGE('',*,*,#1814,.T.);
#2299=ORIENTED_EDGE('',*,*,#1811,.T.);
#2300=ORIENTED_EDGE('',*,*,#1808,.T.);
#2301=ORIENTED_EDGE('',*,*,#1805,.T.);
#2302=ORIENTED_EDGE('',*,*,#1802,.T.);
#2303=ORIENTED_EDGE('',*,*,#1799,.T.);
#2304=ORIENTED_EDGE('',*,*,#1796,.T.);
#2305=ORIENTED_EDGE('',*,*,#1793,.T.);
#2306=ORIENTED_EDGE('',*,*,#1790,.T.);
#2307=ORIENTED_EDGE('',*,*,#1787,.T.);
#2308=ORIENTED_EDGE('',*,*,#1784,.T.);
#2309=ORIENTED_EDGE('',*,*,#1781,.T.);
#2310=ORIENTED_EDGE('',*,*,#1778,.T.);
#2311=ORIENTED_EDGE('',*,*,#1775,.T.);
#2312=ORIENTED_EDGE('',*,*,#1772,.T.);
#2313=ORIENTED_EDGE('',*,*,#1769,.T.);
#2314=ORIENTED_EDGE('',*,*,#1766,.T.);
#2315=ORIENTED_EDGE('',*,*,#1763,.T.);
#2316=ORIENTED_EDGE('',*,*,#1760,.T.);
#2317=ORIENTED_EDGE('',*,*,#1751,.T.);
#2318=ORIENTED_EDGE('',*,*,#1748,.T.);
#2319=ORIENTED_EDGE('',*,*,#1745,.T.);
#2320=ORIENTED_EDGE('',*,*,#1742,.T.);
#2321=ORIENTED_EDGE('',*,*,#1723,.T.);
#2322=ORIENTED_EDGE('',*,*,#1726,.T.);
#2323=ORIENTED_EDGE('',*,*,#1716,.T.);
#2324=ORIENTED_EDGE('',*,*,#1720,.T.);
#2325=ORIENTED_EDGE('',*,*,#1825,.F.);
#2326=ORIENTED_EDGE('',*,*,#1815,.F.);
#2327=ORIENTED_EDGE('',*,*,#1819,.F.);
#2328=ORIENTED_EDGE('',*,*,#1822,.F.);
#2329=ORIENTED_EDGE('',*,*,#1752,.T.);
#2330=ORIENTED_EDGE('',*,*,#1755,.T.);
#2331=ORIENTED_EDGE('',*,*,#1812,.T.);
#2332=ORIENTED_EDGE('',*,*,#1809,.T.);
#2333=ORIENTED_EDGE('',*,*,#1806,.T.);
#2334=ORIENTED_EDGE('',*,*,#1803,.T.);
#2335=ORIENTED_EDGE('',*,*,#1800,.T.);
#2336=ORIENTED_EDGE('',*,*,#1797,.T.);
#2337=ORIENTED_EDGE('',*,*,#1794,.T.);
#2338=ORIENTED_EDGE('',*,*,#1791,.T.);
#2339=ORIENTED_EDGE('',*,*,#1788,.T.);
#2340=ORIENTED_EDGE('',*,*,#1785,.T.);
#2341=ORIENTED_EDGE('',*,*,#1782,.T.);
#2342=ORIENTED_EDGE('',*,*,#1779,.T.);
#2343=ORIENTED_EDGE('',*,*,#1776,.T.);
#2344=ORIENTED_EDGE('',*,*,#1773,.T.);
#2345=ORIENTED_EDGE('',*,*,#1770,.T.);
#2346=ORIENTED_EDGE('',*,*,#1767,.T.);
#2347=ORIENTED_EDGE('',*,*,#1764,.T.);
#2348=ORIENTED_EDGE('',*,*,#1761,.T.);
#2349=ORIENTED_EDGE('',*,*,#1758,.T.);
#2350=ORIENTED_EDGE('',*,*,#1749,.T.);
#2351=ORIENTED_EDGE('',*,*,#1746,.T.);
#2352=ORIENTED_EDGE('',*,*,#1743,.T.);
#2353=ORIENTED_EDGE('',*,*,#1740,.T.);
#2964=PLANE('',#3412);
#2965=PLANE('',#3413);
#2966=PLANE('',#3414);
#2967=PLANE('',#3415);
#2968=PLANE('',#3416);
#2969=PLANE('',#3417);
#2970=PLANE('',#3418);
#2971=PLANE('',#3419);
#2972=PLANE('',#3420);
#2973=PLANE('',#3421);
#2974=PLANE('',#3497);
#2975=PLANE('',#3498);
#2976=PLANE('',#3499);
#2977=PLANE('',#3500);
#2978=PLANE('',#3501);
#2979=PLANE('',#3502);
#3078=ADVANCED_FACE('',(#457),#2964,.F.);
#3079=ADVANCED_FACE('',(#458),#2965,.F.);
#3080=ADVANCED_FACE('',(#459),#2966,.F.);
#3081=ADVANCED_FACE('',(#460),#2967,.F.);
#3082=ADVANCED_FACE('',(#461),#2968,.T.);
#3083=ADVANCED_FACE('',(#462),#2969,.F.);
#3084=ADVANCED_FACE('',(#463),#2970,.F.);
#3085=ADVANCED_FACE('',(#464),#2971,.F.);
#3086=ADVANCED_FACE('',(#465),#2972,.F.);
#3087=ADVANCED_FACE('',(#466),#2973,.T.);
#3088=ADVANCED_FACE('',(#467),#397,.F.);
#3089=ADVANCED_FACE('',(#468),#398,.F.);
#3090=ADVANCED_FACE('',(#469),#399,.F.);
#3091=ADVANCED_FACE('',(#470),#400,.F.);
#3092=ADVANCED_FACE('',(#471),#401,.F.);
#3093=ADVANCED_FACE('',(#472),#402,.F.);
#3094=ADVANCED_FACE('',(#473),#403,.F.);
#3095=ADVANCED_FACE('',(#474),#404,.F.);
#3096=ADVANCED_FACE('',(#475),#405,.F.);
#3097=ADVANCED_FACE('',(#476),#406,.F.);
#3098=ADVANCED_FACE('',(#477),#407,.F.);
#3099=ADVANCED_FACE('',(#478),#408,.F.);
#3100=ADVANCED_FACE('',(#479),#409,.F.);
#3101=ADVANCED_FACE('',(#480),#410,.F.);
#3102=ADVANCED_FACE('',(#481),#411,.F.);
#3103=ADVANCED_FACE('',(#482),#412,.F.);
#3104=ADVANCED_FACE('',(#483),#413,.F.);
#3105=ADVANCED_FACE('',(#484),#414,.F.);
#3106=ADVANCED_FACE('',(#485),#415,.F.);
#3107=ADVANCED_FACE('',(#486),#416,.F.);
#3108=ADVANCED_FACE('',(#487),#417,.F.);
#3109=ADVANCED_FACE('',(#488),#418,.F.);
#3110=ADVANCED_FACE('',(#489),#419,.F.);
#3111=ADVANCED_FACE('',(#490),#420,.F.);
#3112=ADVANCED_FACE('',(#491),#421,.F.);
#3113=ADVANCED_FACE('',(#492),#2974,.T.);
#3114=ADVANCED_FACE('',(#493),#2975,.T.);
#3115=ADVANCED_FACE('',(#494),#2976,.T.);
#3116=ADVANCED_FACE('',(#495),#2977,.T.);
#3117=ADVANCED_FACE('',(#496,#192,#193,#194,#195,#196,#197,#198,#199,#200,
#201,#202,#203,#204,#205,#206,#207,#208,#209,#210,#211,#212,#213,#214,#215,
#216,#217,#218),#2978,.T.);
#3118=ADVANCED_FACE('',(#497,#219,#220,#221,#222,#223,#224,#225,#226,#227,
#228,#229,#230,#231,#232,#233,#234,#235,#236,#237,#238,#239,#240,#241,#242,
#243),#2979,.F.);
#3261=CLOSED_SHELL('',(#3078,#3079,#3080,#3081,#3082,#3083,#3084,#3085,
#3086,#3087,#3088,#3089,#3090,#3091,#3092,#3093,#3094,#3095,#3096,#3097,
#3098,#3099,#3100,#3101,#3102,#3103,#3104,#3105,#3106,#3107,#3108,#3109,
#3110,#3111,#3112,#3113,#3114,#3115,#3116,#3117,#3118));
#3411=AXIS2_PLACEMENT_3D('',#4743,#3765,#3766);
#3412=AXIS2_PLACEMENT_3D('',#4744,#3767,#3768);
#3413=AXIS2_PLACEMENT_3D('',#4753,#3773,#3774);
#3414=AXIS2_PLACEMENT_3D('',#4759,#3778,#3779);
#3415=AXIS2_PLACEMENT_3D('',#4765,#3783,#3784);
#3416=AXIS2_PLACEMENT_3D('',#4768,#3787,#3788);
#3417=AXIS2_PLACEMENT_3D('',#4769,#3789,#3790);
#3418=AXIS2_PLACEMENT_3D('',#4778,#3795,#3796);
#3419=AXIS2_PLACEMENT_3D('',#4784,#3800,#3801);
#3420=AXIS2_PLACEMENT_3D('',#4790,#3805,#3806);
#3421=AXIS2_PLACEMENT_3D('',#4793,#3809,#3810);
#3422=AXIS2_PLACEMENT_3D('',#4794,#3811,#3812);
#3423=AXIS2_PLACEMENT_3D('',#4796,#3813,#3814);
#3424=AXIS2_PLACEMENT_3D('',#4799,#3816,#3817);
#3425=AXIS2_PLACEMENT_3D('',#4800,#3818,#3819);
#3426=AXIS2_PLACEMENT_3D('',#4802,#3820,#3821);
#3427=AXIS2_PLACEMENT_3D('',#4805,#3823,#3824);
#3428=AXIS2_PLACEMENT_3D('',#4806,#3825,#3826);
#3429=AXIS2_PLACEMENT_3D('',#4808,#3827,#3828);
#3430=AXIS2_PLACEMENT_3D('',#4811,#3830,#3831);
#3431=AXIS2_PLACEMENT_3D('',#4812,#3832,#3833);
#3432=AXIS2_PLACEMENT_3D('',#4814,#3834,#3835);
#3433=AXIS2_PLACEMENT_3D('',#4817,#3837,#3838);
#3434=AXIS2_PLACEMENT_3D('',#4818,#3839,#3840);
#3435=AXIS2_PLACEMENT_3D('',#4820,#3841,#3842);
#3436=AXIS2_PLACEMENT_3D('',#4823,#3844,#3845);
#3437=AXIS2_PLACEMENT_3D('',#4824,#3846,#3847);
#3438=AXIS2_PLACEMENT_3D('',#4826,#3848,#3849);
#3439=AXIS2_PLACEMENT_3D('',#4829,#3851,#3852);
#3440=AXIS2_PLACEMENT_3D('',#4830,#3853,#3854);
#3441=AXIS2_PLACEMENT_3D('',#4832,#3855,#3856);
#3442=AXIS2_PLACEMENT_3D('',#4835,#3858,#3859);
#3443=AXIS2_PLACEMENT_3D('',#4836,#3860,#3861);
#3444=AXIS2_PLACEMENT_3D('',#4838,#3862,#3863);
#3445=AXIS2_PLACEMENT_3D('',#4841,#3865,#3866);
#3446=AXIS2_PLACEMENT_3D('',#4842,#3867,#3868);
#3447=AXIS2_PLACEMENT_3D('',#4844,#3869,#3870);
#3448=AXIS2_PLACEMENT_3D('',#4847,#3872,#3873);
#3449=AXIS2_PLACEMENT_3D('',#4848,#3874,#3875);
#3450=AXIS2_PLACEMENT_3D('',#4850,#3876,#3877);
#3451=AXIS2_PLACEMENT_3D('',#4853,#3879,#3880);
#3452=AXIS2_PLACEMENT_3D('',#4854,#3881,#3882);
#3453=AXIS2_PLACEMENT_3D('',#4856,#3883,#3884);
#3454=AXIS2_PLACEMENT_3D('',#4859,#3886,#3887);
#3455=AXIS2_PLACEMENT_3D('',#4860,#3888,#3889);
#3456=AXIS2_PLACEMENT_3D('',#4862,#3890,#3891);
#3457=AXIS2_PLACEMENT_3D('',#4865,#3893,#3894);
#3458=AXIS2_PLACEMENT_3D('',#4866,#3895,#3896);
#3459=AXIS2_PLACEMENT_3D('',#4868,#3897,#3898);
#3460=AXIS2_PLACEMENT_3D('',#4871,#3900,#3901);
#3461=AXIS2_PLACEMENT_3D('',#4872,#3902,#3903);
#3462=AXIS2_PLACEMENT_3D('',#4874,#3904,#3905);
#3463=AXIS2_PLACEMENT_3D('',#4877,#3907,#3908);
#3464=AXIS2_PLACEMENT_3D('',#4878,#3909,#3910);
#3465=AXIS2_PLACEMENT_3D('',#4880,#3911,#3912);
#3466=AXIS2_PLACEMENT_3D('',#4883,#3914,#3915);
#3467=AXIS2_PLACEMENT_3D('',#4884,#3916,#3917);
#3468=AXIS2_PLACEMENT_3D('',#4886,#3918,#3919);
#3469=AXIS2_PLACEMENT_3D('',#4889,#3921,#3922);
#3470=AXIS2_PLACEMENT_3D('',#4890,#3923,#3924);
#3471=AXIS2_PLACEMENT_3D('',#4892,#3925,#3926);
#3472=AXIS2_PLACEMENT_3D('',#4895,#3928,#3929);
#3473=AXIS2_PLACEMENT_3D('',#4896,#3930,#3931);
#3474=AXIS2_PLACEMENT_3D('',#4898,#3932,#3933);
#3475=AXIS2_PLACEMENT_3D('',#4901,#3935,#3936);
#3476=AXIS2_PLACEMENT_3D('',#4902,#3937,#3938);
#3477=AXIS2_PLACEMENT_3D('',#4904,#3939,#3940);
#3478=AXIS2_PLACEMENT_3D('',#4907,#3942,#3943);
#3479=AXIS2_PLACEMENT_3D('',#4908,#3944,#3945);
#3480=AXIS2_PLACEMENT_3D('',#4910,#3946,#3947);
#3481=AXIS2_PLACEMENT_3D('',#4913,#3949,#3950);
#3482=AXIS2_PLACEMENT_3D('',#4914,#3951,#3952);
#3483=AXIS2_PLACEMENT_3D('',#4916,#3953,#3954);
#3484=AXIS2_PLACEMENT_3D('',#4919,#3956,#3957);
#3485=AXIS2_PLACEMENT_3D('',#4920,#3958,#3959);
#3486=AXIS2_PLACEMENT_3D('',#4922,#3960,#3961);
#3487=AXIS2_PLACEMENT_3D('',#4925,#3963,#3964);
#3488=AXIS2_PLACEMENT_3D('',#4926,#3965,#3966);
#3489=AXIS2_PLACEMENT_3D('',#4928,#3967,#3968);
#3490=AXIS2_PLACEMENT_3D('',#4931,#3970,#3971);
#3491=AXIS2_PLACEMENT_3D('',#4932,#3972,#3973);
#3492=AXIS2_PLACEMENT_3D('',#4934,#3974,#3975);
#3493=AXIS2_PLACEMENT_3D('',#4937,#3977,#3978);
#3494=AXIS2_PLACEMENT_3D('',#4938,#3979,#3980);
#3495=AXIS2_PLACEMENT_3D('',#4940,#3981,#3982);
#3496=AXIS2_PLACEMENT_3D('',#4943,#3984,#3985);
#3497=AXIS2_PLACEMENT_3D('',#4944,#3986,#3987);
#3498=AXIS2_PLACEMENT_3D('',#4953,#3992,#3993);
#3499=AXIS2_PLACEMENT_3D('',#4959,#3997,#3998);
#3500=AXIS2_PLACEMENT_3D('',#4965,#4002,#4003);
#3501=AXIS2_PLACEMENT_3D('',#4968,#4006,#4007);
#3502=AXIS2_PLACEMENT_3D('',#4969,#4008,#4009);
#3765=DIRECTION('axis',(0.,0.,1.));
#3766=DIRECTION('refdir',(1.,0.,0.));
#3767=DIRECTION('center_axis',(0.,-1.,0.));
#3768=DIRECTION('ref_axis',(1.,0.,0.));
#3769=DIRECTION('',(-1.,0.,0.));
#3770=DIRECTION('',(0.,0.,1.));
#3771=DIRECTION('',(1.,0.,0.));
#3772=DIRECTION('',(0.,0.,1.));
#3773=DIRECTION('center_axis',(-1.,0.,0.));
#3774=DIRECTION('ref_axis',(0.,-1.,0.));
#3775=DIRECTION('',(0.,1.,0.));
#3776=DIRECTION('',(0.,-1.,0.));
#3777=DIRECTION('',(0.,0.,1.));
#3778=DIRECTION('center_axis',(0.,1.,0.));
#3779=DIRECTION('ref_axis',(-1.,0.,0.));
#3780=DIRECTION('',(1.,0.,0.));
#3781=DIRECTION('',(-1.,0.,0.));
#3782=DIRECTION('',(0.,0.,1.));
#3783=DIRECTION('center_axis',(1.,0.,0.));
#3784=DIRECTION('ref_axis',(0.,1.,0.));
#3785=DIRECTION('',(0.,-1.,0.));
#3786=DIRECTION('',(0.,1.,0.));
#3787=DIRECTION('center_axis',(0.,0.,1.));
#3788=DIRECTION('ref_axis',(1.,0.,0.));
#3789=DIRECTION('center_axis',(0.,-1.,0.));
#3790=DIRECTION('ref_axis',(1.,0.,0.));
#3791=DIRECTION('',(-1.,0.,0.));
#3792=DIRECTION('',(0.,0.,1.));
#3793=DIRECTION('',(1.,0.,0.));
#3794=DIRECTION('',(0.,0.,1.));
#3795=DIRECTION('center_axis',(-1.,0.,0.));
#3796=DIRECTION('ref_axis',(0.,-1.,0.));
#3797=DIRECTION('',(0.,1.,0.));
#3798=DIRECTION('',(0.,-1.,0.));
#3799=DIRECTION('',(0.,0.,1.));
#3800=DIRECTION('center_axis',(0.,1.,0.));
#3801=DIRECTION('ref_axis',(-1.,0.,0.));
#3802=DIRECTION('',(1.,0.,0.));
#3803=DIRECTION('',(-1.,0.,0.));
#3804=DIRECTION('',(0.,0.,1.));
#3805=DIRECTION('center_axis',(1.,0.,0.));
#3806=DIRECTION('ref_axis',(0.,1.,0.));
#3807=DIRECTION('',(0.,-1.,0.));
#3808=DIRECTION('',(0.,1.,0.));
#3809=DIRECTION('center_axis',(0.,0.,1.));
#3810=DIRECTION('ref_axis',(1.,0.,0.));
#3811=DIRECTION('center_axis',(0.,0.,1.));
#3812=DIRECTION('ref_axis',(1.,0.,0.));
#3813=DIRECTION('center_axis',(0.,0.,1.));
#3814=DIRECTION('ref_axis',(1.,0.,0.));
#3815=DIRECTION('',(0.,0.,1.));
#3816=DIRECTION('center_axis',(0.,0.,-1.));
#3817=DIRECTION('ref_axis',(1.,0.,0.));
#3818=DIRECTION('center_axis',(0.,0.,1.));
#3819=DIRECTION('ref_axis',(1.,0.,0.));
#3820=DIRECTION('center_axis',(0.,0.,1.));
#3821=DIRECTION('ref_axis',(1.,0.,0.));
#3822=DIRECTION('',(0.,0.,1.));
#3823=DIRECTION('center_axis',(0.,0.,-1.));
#3824=DIRECTION('ref_axis',(1.,0.,0.));
#3825=DIRECTION('center_axis',(0.,0.,1.));
#3826=DIRECTION('ref_axis',(1.,0.,0.));
#3827=DIRECTION('center_axis',(0.,0.,1.));
#3828=DIRECTION('ref_axis',(1.,0.,0.));
#3829=DIRECTION('',(0.,0.,1.));
#3830=DIRECTION('center_axis',(0.,0.,-1.));
#3831=DIRECTION('ref_axis',(1.,0.,0.));
#3832=DIRECTION('center_axis',(0.,0.,1.));
#3833=DIRECTION('ref_axis',(1.,0.,0.));
#3834=DIRECTION('center_axis',(0.,0.,1.));
#3835=DIRECTION('ref_axis',(1.,0.,0.));
#3836=DIRECTION('',(0.,0.,1.));
#3837=DIRECTION('center_axis',(0.,0.,-1.));
#3838=DIRECTION('ref_axis',(1.,0.,0.));
#3839=DIRECTION('center_axis',(0.,0.,1.));
#3840=DIRECTION('ref_axis',(1.,0.,0.));
#3841=DIRECTION('center_axis',(0.,0.,1.));
#3842=DIRECTION('ref_axis',(1.,0.,0.));
#3843=DIRECTION('',(0.,0.,1.));
#3844=DIRECTION('center_axis',(0.,0.,-1.));
#3845=DIRECTION('ref_axis',(1.,0.,0.));
#3846=DIRECTION('center_axis',(0.,0.,1.));
#3847=DIRECTION('ref_axis',(1.,0.,0.));
#3848=DIRECTION('center_axis',(0.,0.,1.));
#3849=DIRECTION('ref_axis',(1.,0.,0.));
#3850=DIRECTION('',(0.,0.,1.));
#3851=DIRECTION('center_axis',(0.,0.,-1.));
#3852=DIRECTION('ref_axis',(1.,0.,0.));
#3853=DIRECTION('center_axis',(0.,0.,1.));
#3854=DIRECTION('ref_axis',(1.,0.,0.));
#3855=DIRECTION('center_axis',(0.,0.,1.));
#3856=DIRECTION('ref_axis',(1.,0.,0.));
#3857=DIRECTION('',(0.,0.,1.));
#3858=DIRECTION('center_axis',(0.,0.,-1.));
#3859=DIRECTION('ref_axis',(1.,0.,0.));
#3860=DIRECTION('center_axis',(0.,0.,1.));
#3861=DIRECTION('ref_axis',(1.,0.,0.));
#3862=DIRECTION('center_axis',(0.,0.,1.));
#3863=DIRECTION('ref_axis',(1.,0.,0.));
#3864=DIRECTION('',(0.,0.,1.));
#3865=DIRECTION('center_axis',(0.,0.,-1.));
#3866=DIRECTION('ref_axis',(1.,0.,0.));
#3867=DIRECTION('center_axis',(0.,0.,1.));
#3868=DIRECTION('ref_axis',(1.,0.,0.));
#3869=DIRECTION('center_axis',(0.,0.,1.));
#3870=DIRECTION('ref_axis',(1.,0.,0.));
#3871=DIRECTION('',(0.,0.,1.));
#3872=DIRECTION('center_axis',(0.,0.,-1.));
#3873=DIRECTION('ref_axis',(1.,0.,0.));
#3874=DIRECTION('center_axis',(0.,0.,1.));
#3875=DIRECTION('ref_axis',(1.,0.,0.));
#3876=DIRECTION('center_axis',(0.,0.,1.));
#3877=DIRECTION('ref_axis',(1.,0.,0.));
#3878=DIRECTION('',(0.,0.,1.));
#3879=DIRECTION('center_axis',(0.,0.,-1.));
#3880=DIRECTION('ref_axis',(1.,0.,0.));
#3881=DIRECTION('center_axis',(0.,0.,1.));
#3882=DIRECTION('ref_axis',(1.,0.,0.));
#3883=DIRECTION('center_axis',(0.,0.,1.));
#3884=DIRECTION('ref_axis',(1.,0.,0.));
#3885=DIRECTION('',(0.,0.,1.));
#3886=DIRECTION('center_axis',(0.,0.,-1.));
#3887=DIRECTION('ref_axis',(1.,0.,0.));
#3888=DIRECTION('center_axis',(0.,0.,1.));
#3889=DIRECTION('ref_axis',(1.,0.,0.));
#3890=DIRECTION('center_axis',(0.,0.,1.));
#3891=DIRECTION('ref_axis',(1.,0.,0.));
#3892=DIRECTION('',(0.,0.,1.));
#3893=DIRECTION('center_axis',(0.,0.,-1.));
#3894=DIRECTION('ref_axis',(1.,0.,0.));
#3895=DIRECTION('center_axis',(0.,0.,1.));
#3896=DIRECTION('ref_axis',(1.,0.,0.));
#3897=DIRECTION('center_axis',(0.,0.,1.));
#3898=DIRECTION('ref_axis',(1.,0.,0.));
#3899=DIRECTION('',(0.,0.,1.));
#3900=DIRECTION('center_axis',(0.,0.,-1.));
#3901=DIRECTION('ref_axis',(1.,0.,0.));
#3902=DIRECTION('center_axis',(0.,0.,1.));
#3903=DIRECTION('ref_axis',(1.,0.,0.));
#3904=DIRECTION('center_axis',(0.,0.,1.));
#3905=DIRECTION('ref_axis',(1.,0.,0.));
#3906=DIRECTION('',(0.,0.,1.));
#3907=DIRECTION('center_axis',(0.,0.,-1.));
#3908=DIRECTION('ref_axis',(1.,0.,0.));
#3909=DIRECTION('center_axis',(0.,0.,1.));
#3910=DIRECTION('ref_axis',(1.,0.,0.));
#3911=DIRECTION('center_axis',(0.,0.,1.));
#3912=DIRECTION('ref_axis',(1.,0.,0.));
#3913=DIRECTION('',(0.,0.,1.));
#3914=DIRECTION('center_axis',(0.,0.,-1.));
#3915=DIRECTION('ref_axis',(1.,0.,0.));
#3916=DIRECTION('center_axis',(0.,0.,1.));
#3917=DIRECTION('ref_axis',(1.,0.,0.));
#3918=DIRECTION('center_axis',(0.,0.,1.));
#3919=DIRECTION('ref_axis',(1.,0.,0.));
#3920=DIRECTION('',(0.,0.,1.));
#3921=DIRECTION('center_axis',(0.,0.,-1.));
#3922=DIRECTION('ref_axis',(1.,0.,0.));
#3923=DIRECTION('center_axis',(0.,0.,1.));
#3924=DIRECTION('ref_axis',(1.,0.,0.));
#3925=DIRECTION('center_axis',(0.,0.,1.));
#3926=DIRECTION('ref_axis',(1.,0.,0.));
#3927=DIRECTION('',(0.,0.,1.));
#3928=DIRECTION('center_axis',(0.,0.,-1.));
#3929=DIRECTION('ref_axis',(1.,0.,0.));
#3930=DIRECTION('center_axis',(0.,0.,1.));
#3931=DIRECTION('ref_axis',(1.,0.,0.));
#3932=DIRECTION('center_axis',(0.,0.,1.));
#3933=DIRECTION('ref_axis',(1.,0.,0.));
#3934=DIRECTION('',(0.,0.,1.));
#3935=DIRECTION('center_axis',(0.,0.,-1.));
#3936=DIRECTION('ref_axis',(1.,0.,0.));
#3937=DIRECTION('center_axis',(0.,0.,1.));
#3938=DIRECTION('ref_axis',(1.,0.,0.));
#3939=DIRECTION('center_axis',(0.,0.,1.));
#3940=DIRECTION('ref_axis',(1.,0.,0.));
#3941=DIRECTION('',(0.,0.,1.));
#3942=DIRECTION('center_axis',(0.,0.,-1.));
#3943=DIRECTION('ref_axis',(1.,0.,0.));
#3944=DIRECTION('center_axis',(0.,0.,1.));
#3945=DIRECTION('ref_axis',(1.,0.,0.));
#3946=DIRECTION('center_axis',(0.,0.,1.));
#3947=DIRECTION('ref_axis',(1.,0.,0.));
#3948=DIRECTION('',(0.,0.,1.));
#3949=DIRECTION('center_axis',(0.,0.,-1.));
#3950=DIRECTION('ref_axis',(1.,0.,0.));
#3951=DIRECTION('center_axis',(0.,0.,1.));
#3952=DIRECTION('ref_axis',(1.,0.,0.));
#3953=DIRECTION('center_axis',(0.,0.,1.));
#3954=DIRECTION('ref_axis',(1.,0.,0.));
#3955=DIRECTION('',(0.,0.,1.));
#3956=DIRECTION('center_axis',(0.,0.,-1.));
#3957=DIRECTION('ref_axis',(1.,0.,0.));
#3958=DIRECTION('center_axis',(0.,0.,1.));
#3959=DIRECTION('ref_axis',(1.,0.,0.));
#3960=DIRECTION('center_axis',(0.,0.,1.));
#3961=DIRECTION('ref_axis',(1.,0.,0.));
#3962=DIRECTION('',(0.,0.,1.));
#3963=DIRECTION('center_axis',(0.,0.,-1.));
#3964=DIRECTION('ref_axis',(1.,0.,0.));
#3965=DIRECTION('center_axis',(0.,0.,1.));
#3966=DIRECTION('ref_axis',(1.,0.,0.));
#3967=DIRECTION('center_axis',(0.,0.,1.));
#3968=DIRECTION('ref_axis',(1.,0.,0.));
#3969=DIRECTION('',(0.,0.,1.));
#3970=DIRECTION('center_axis',(0.,0.,-1.));
#3971=DIRECTION('ref_axis',(1.,0.,0.));
#3972=DIRECTION('center_axis',(0.,0.,1.));
#3973=DIRECTION('ref_axis',(1.,0.,0.));
#3974=DIRECTION('center_axis',(0.,0.,1.));
#3975=DIRECTION('ref_axis',(1.,0.,0.));
#3976=DIRECTION('',(0.,0.,1.));
#3977=DIRECTION('center_axis',(0.,0.,-1.));
#3978=DIRECTION('ref_axis',(1.,0.,0.));
#3979=DIRECTION('center_axis',(0.,0.,1.));
#3980=DIRECTION('ref_axis',(1.,0.,0.));
#3981=DIRECTION('center_axis',(0.,0.,1.));
#3982=DIRECTION('ref_axis',(1.,0.,0.));
#3983=DIRECTION('',(0.,0.,1.));
#3984=DIRECTION('center_axis',(0.,0.,-1.));
#3985=DIRECTION('ref_axis',(1.,0.,0.));
#3986=DIRECTION('center_axis',(0.,1.,0.));
#3987=DIRECTION('ref_axis',(-1.,0.,0.));
#3988=DIRECTION('',(-1.,0.,0.));
#3989=DIRECTION('',(0.,0.,1.));
#3990=DIRECTION('',(-1.,0.,0.));
#3991=DIRECTION('',(0.,0.,1.));
#3992=DIRECTION('center_axis',(1.,0.,0.));
#3993=DIRECTION('ref_axis',(0.,1.,0.));
#3994=DIRECTION('',(0.,1.,0.));
#3995=DIRECTION('',(0.,1.,0.));
#3996=DIRECTION('',(0.,0.,1.));
#3997=DIRECTION('center_axis',(0.,-1.,0.));
#3998=DIRECTION('ref_axis',(1.,0.,0.));
#3999=DIRECTION('',(1.,0.,0.));
#4000=DIRECTION('',(1.,0.,0.));
#4001=DIRECTION('',(0.,0.,1.));
#4002=DIRECTION('center_axis',(-1.,0.,0.));
#4003=DIRECTION('ref_axis',(0.,-1.,0.));
#4004=DIRECTION('',(0.,-1.,0.));
#4005=DIRECTION('',(0.,-1.,0.));
#4006=DIRECTION('center_axis',(0.,0.,1.));
#4007=DIRECTION('ref_axis',(1.,0.,0.));
#4008=DIRECTION('center_axis',(0.,0.,1.));
#4009=DIRECTION('ref_axis',(1.,0.,0.));
#4743=CARTESIAN_POINT('',(0.,0.,0.));
#4744=CARTESIAN_POINT('Origin',(9.5,-0.3,0.7));
#4745=CARTESIAN_POINT('',(11.5,-0.3,1.));
#4746=CARTESIAN_POINT('',(9.5,-0.3,1.));
#4747=CARTESIAN_POINT('',(8.5,-0.3,1.));
#4748=CARTESIAN_POINT('',(11.5,-0.3,0.7));
#4749=CARTESIAN_POINT('',(11.5,-0.3,0.7));
#4750=CARTESIAN_POINT('',(9.5,-0.3,0.7));
#4751=CARTESIAN_POINT('',(9.5,-0.3,0.7));
#4752=CARTESIAN_POINT('',(9.5,-0.3,0.7));
#4753=CARTESIAN_POINT('Origin',(9.5,0.3,0.7));
#4754=CARTESIAN_POINT('',(9.5,0.3,1.));
#4755=CARTESIAN_POINT('',(9.5,0.15,1.));
#4756=CARTESIAN_POINT('',(9.5,0.3,0.7));
#4757=CARTESIAN_POINT('',(9.5,0.3,0.7));
#4758=CARTESIAN_POINT('',(9.5,0.3,0.7));
#4759=CARTESIAN_POINT('Origin',(11.5,0.3,0.7));
#4760=CARTESIAN_POINT('',(11.5,0.3,1.));
#4761=CARTESIAN_POINT('',(9.5,0.3,1.));
#4762=CARTESIAN_POINT('',(11.5,0.3,0.7));
#4763=CARTESIAN_POINT('',(11.5,0.3,0.7));
#4764=CARTESIAN_POINT('',(11.5,0.3,0.7));
#4765=CARTESIAN_POINT('Origin',(11.5,-0.3,0.7));
#4766=CARTESIAN_POINT('',(11.5,-0.15,1.));
#4767=CARTESIAN_POINT('',(11.5,-0.3,0.7));
#4768=CARTESIAN_POINT('Origin',(10.5,0.,0.7));
#4769=CARTESIAN_POINT('Origin',(3.5,-0.3,0.7));
#4770=CARTESIAN_POINT('',(5.5,-0.3,1.));
#4771=CARTESIAN_POINT('',(3.5,-0.3,1.));
#4772=CARTESIAN_POINT('',(5.5,-0.3,1.));
#4773=CARTESIAN_POINT('',(5.5,-0.3,0.7));
#4774=CARTESIAN_POINT('',(5.5,-0.3,0.7));
#4775=CARTESIAN_POINT('',(3.5,-0.3,0.7));
#4776=CARTESIAN_POINT('',(3.5,-0.3,0.7));
#4777=CARTESIAN_POINT('',(3.5,-0.3,0.7));
#4778=CARTESIAN_POINT('Origin',(3.5,0.3,0.7));
#4779=CARTESIAN_POINT('',(3.5,0.3,1.));
#4780=CARTESIAN_POINT('',(3.5,0.15,1.));
#4781=CARTESIAN_POINT('',(3.5,0.3,0.7));
#4782=CARTESIAN_POINT('',(3.5,0.3,0.7));
#4783=CARTESIAN_POINT('',(3.5,0.3,0.7));
#4784=CARTESIAN_POINT('Origin',(5.5,0.3,0.7));
#4785=CARTESIAN_POINT('',(5.5,0.3,1.));
#4786=CARTESIAN_POINT('',(6.5,0.3,1.));
#4787=CARTESIAN_POINT('',(5.5,0.3,0.7));
#4788=CARTESIAN_POINT('',(5.5,0.3,0.7));
#4789=CARTESIAN_POINT('',(5.5,0.3,0.7));
#4790=CARTESIAN_POINT('Origin',(5.5,-0.3,0.7));
#4791=CARTESIAN_POINT('',(5.5,-0.15,1.));
#4792=CARTESIAN_POINT('',(5.5,-0.3,0.7));
#4793=CARTESIAN_POINT('Origin',(4.5,0.,0.7));
#4794=CARTESIAN_POINT('Origin',(10.5,-2.5,-0.1));
#4795=CARTESIAN_POINT('',(10.25,-2.5,0.));
#4796=CARTESIAN_POINT('Origin',(10.5,-2.5,0.));
#4797=CARTESIAN_POINT('',(10.25,-2.5,1.));
#4798=CARTESIAN_POINT('',(10.25,-2.5,-0.1));
#4799=CARTESIAN_POINT('Origin',(10.5,-2.5,1.));
#4800=CARTESIAN_POINT('Origin',(4.5,2.5,-0.1));
#4801=CARTESIAN_POINT('',(4.25,2.5,0.));
#4802=CARTESIAN_POINT('Origin',(4.5,2.5,0.));
#4803=CARTESIAN_POINT('',(4.25,2.5,1.));
#4804=CARTESIAN_POINT('',(4.25,2.5,-0.1));
#4805=CARTESIAN_POINT('Origin',(4.5,2.5,1.));
#4806=CARTESIAN_POINT('Origin',(4.5,-2.5,-0.1));
#4807=CARTESIAN_POINT('',(4.25,-2.5,0.));
#4808=CARTESIAN_POINT('Origin',(4.5,-2.5,0.));
#4809=CARTESIAN_POINT('',(4.25,-2.5,1.));
#4810=CARTESIAN_POINT('',(4.25,-2.5,-0.1));
#4811=CARTESIAN_POINT('Origin',(4.5,-2.5,1.));
#4812=CARTESIAN_POINT('Origin',(10.5,2.5,-0.1));
#4813=CARTESIAN_POINT('',(10.25,2.5,0.));
#4814=CARTESIAN_POINT('Origin',(10.5,2.5,0.));
#4815=CARTESIAN_POINT('',(10.25,2.5,1.));
#4816=CARTESIAN_POINT('',(10.25,2.5,-0.1));
#4817=CARTESIAN_POINT('Origin',(10.5,2.5,1.));
#4818=CARTESIAN_POINT('Origin',(7.5,-4.,-0.1));
#4819=CARTESIAN_POINT('',(7.16,-4.,0.));
#4820=CARTESIAN_POINT('Origin',(7.5,-4.,0.));
#4821=CARTESIAN_POINT('',(7.16,-4.,1.));
#4822=CARTESIAN_POINT('',(7.16,-4.,-0.1));
#4823=CARTESIAN_POINT('Origin',(7.5,-4.,1.));
#4824=CARTESIAN_POINT('Origin',(7.5,4.,-0.1));
#4825=CARTESIAN_POINT('',(7.16,4.,0.));
#4826=CARTESIAN_POINT('Origin',(7.5,4.,0.));
#4827=CARTESIAN_POINT('',(7.16,4.,1.));
#4828=CARTESIAN_POINT('',(7.16,4.,-0.1));
#4829=CARTESIAN_POINT('Origin',(7.5,4.,1.));
#4830=CARTESIAN_POINT('Origin',(12.5,2.5,-0.1));
#4831=CARTESIAN_POINT('',(12.16,2.5,0.));
#4832=CARTESIAN_POINT('Origin',(12.5,2.5,0.));
#4833=CARTESIAN_POINT('',(12.16,2.5,1.));
#4834=CARTESIAN_POINT('',(12.16,2.5,-0.1));
#4835=CARTESIAN_POINT('Origin',(12.5,2.5,1.));
#4836=CARTESIAN_POINT('Origin',(12.5,-2.5,-0.1));
#4837=CARTESIAN_POINT('',(12.16,-2.5,0.));
#4838=CARTESIAN_POINT('Origin',(12.5,-2.5,0.));
#4839=CARTESIAN_POINT('',(12.16,-2.5,1.));
#4840=CARTESIAN_POINT('',(12.16,-2.5,-0.1));
#4841=CARTESIAN_POINT('Origin',(12.5,-2.5,1.));
#4842=CARTESIAN_POINT('Origin',(10.,5.,-0.1));
#4843=CARTESIAN_POINT('',(9.66,5.,0.));
#4844=CARTESIAN_POINT('Origin',(10.,5.,0.));
#4845=CARTESIAN_POINT('',(9.66,5.,1.));
#4846=CARTESIAN_POINT('',(9.66,5.,-0.1));
#4847=CARTESIAN_POINT('Origin',(10.,5.,1.));
#4848=CARTESIAN_POINT('Origin',(7.5,5.,-0.1));
#4849=CARTESIAN_POINT('',(7.16,5.,0.));
#4850=CARTESIAN_POINT('Origin',(7.5,5.,0.));
#4851=CARTESIAN_POINT('',(7.16,5.,1.));
#4852=CARTESIAN_POINT('',(7.16,5.,-0.1));
#4853=CARTESIAN_POINT('Origin',(7.5,5.,1.));
#4854=CARTESIAN_POINT('Origin',(2.5,-5.,-0.1));
#4855=CARTESIAN_POINT('',(2.16,-5.,0.));
#4856=CARTESIAN_POINT('Origin',(2.5,-5.,0.));
#4857=CARTESIAN_POINT('',(2.16,-5.,1.));
#4858=CARTESIAN_POINT('',(2.16,-5.,-0.1));
#4859=CARTESIAN_POINT('Origin',(2.5,-5.,1.));
#4860=CARTESIAN_POINT('Origin',(7.5,-2.5,-0.1));
#4861=CARTESIAN_POINT('',(7.16,-2.5,0.));
#4862=CARTESIAN_POINT('Origin',(7.5,-2.5,0.));
#4863=CARTESIAN_POINT('',(7.16,-2.5,1.));
#4864=CARTESIAN_POINT('',(7.16,-2.5,-0.1));
#4865=CARTESIAN_POINT('Origin',(7.5,-2.5,1.));
#4866=CARTESIAN_POINT('Origin',(5.,5.,-0.1));
#4867=CARTESIAN_POINT('',(4.66,5.,0.));
#4868=CARTESIAN_POINT('Origin',(5.,5.,0.));
#4869=CARTESIAN_POINT('',(4.66,5.,1.));
#4870=CARTESIAN_POINT('',(4.66,5.,-0.1));
#4871=CARTESIAN_POINT('Origin',(5.,5.,1.));
#4872=CARTESIAN_POINT('Origin',(2.5,5.,-0.1));
#4873=CARTESIAN_POINT('',(2.16,5.,0.));
#4874=CARTESIAN_POINT('Origin',(2.5,5.,0.));
#4875=CARTESIAN_POINT('',(2.16,5.,1.));
#4876=CARTESIAN_POINT('',(2.16,5.,-0.1));
#4877=CARTESIAN_POINT('Origin',(2.5,5.,1.));
#4878=CARTESIAN_POINT('Origin',(2.5,0.,-0.1));
#4879=CARTESIAN_POINT('',(2.16,-4.163799117101E-17,0.));
#4880=CARTESIAN_POINT('Origin',(2.5,0.,0.));
#4881=CARTESIAN_POINT('',(2.16,4.163799117101E-17,1.));
#4882=CARTESIAN_POINT('',(2.16,-4.163799117101E-17,-0.1));
#4883=CARTESIAN_POINT('Origin',(2.5,0.,1.));
#4884=CARTESIAN_POINT('Origin',(2.5,-2.5,-0.1));
#4885=CARTESIAN_POINT('',(2.16,-2.5,0.));
#4886=CARTESIAN_POINT('Origin',(2.5,-2.5,0.));
#4887=CARTESIAN_POINT('',(2.16,-2.5,1.));
#4888=CARTESIAN_POINT('',(2.16,-2.5,-0.1));
#4889=CARTESIAN_POINT('Origin',(2.5,-2.5,1.));
#4890=CARTESIAN_POINT('Origin',(2.5,2.5,-0.1));
#4891=CARTESIAN_POINT('',(2.16,2.5,0.));
#4892=CARTESIAN_POINT('Origin',(2.5,2.5,0.));
#4893=CARTESIAN_POINT('',(2.16,2.5,1.));
#4894=CARTESIAN_POINT('',(2.16,2.5,-0.1));
#4895=CARTESIAN_POINT('Origin',(2.5,2.5,1.));
#4896=CARTESIAN_POINT('Origin',(5.,-5.,-0.1));
#4897=CARTESIAN_POINT('',(4.66,-5.,0.));
#4898=CARTESIAN_POINT('Origin',(5.,-5.,0.));
#4899=CARTESIAN_POINT('',(4.66,-5.,1.));
#4900=CARTESIAN_POINT('',(4.66,-5.,-0.1));
#4901=CARTESIAN_POINT('Origin',(5.,-5.,1.));
#4902=CARTESIAN_POINT('Origin',(7.5,-5.,-0.1));
#4903=CARTESIAN_POINT('',(7.16,-5.,0.));
#4904=CARTESIAN_POINT('Origin',(7.5,-5.,0.));
#4905=CARTESIAN_POINT('',(7.16,-5.,1.));
#4906=CARTESIAN_POINT('',(7.16,-5.,-0.1));
#4907=CARTESIAN_POINT('Origin',(7.5,-5.,1.));
#4908=CARTESIAN_POINT('Origin',(7.5,0.,-0.1));
#4909=CARTESIAN_POINT('',(7.16,-4.163799117101E-17,0.));
#4910=CARTESIAN_POINT('Origin',(7.5,0.,0.));
#4911=CARTESIAN_POINT('',(7.16,4.163799117101E-17,1.));
#4912=CARTESIAN_POINT('',(7.16,-4.163799117101E-17,-0.1));
#4913=CARTESIAN_POINT('Origin',(7.5,0.,1.));
#4914=CARTESIAN_POINT('Origin',(7.5,2.5,-0.1));
#4915=CARTESIAN_POINT('',(7.16,2.5,0.));
#4916=CARTESIAN_POINT('Origin',(7.5,2.5,0.));
#4917=CARTESIAN_POINT('',(7.16,2.5,1.));
#4918=CARTESIAN_POINT('',(7.16,2.5,-0.1));
#4919=CARTESIAN_POINT('Origin',(7.5,2.5,1.));
#4920=CARTESIAN_POINT('Origin',(10.,-5.,-0.1));
#4921=CARTESIAN_POINT('',(9.66,-5.,0.));
#4922=CARTESIAN_POINT('Origin',(10.,-5.,0.));
#4923=CARTESIAN_POINT('',(9.66,-5.,1.));
#4924=CARTESIAN_POINT('',(9.66,-5.,-0.1));
#4925=CARTESIAN_POINT('Origin',(10.,-5.,1.));
#4926=CARTESIAN_POINT('Origin',(12.5,-5.,-0.1));
#4927=CARTESIAN_POINT('',(12.16,-5.,0.));
#4928=CARTESIAN_POINT('Origin',(12.5,-5.,0.));
#4929=CARTESIAN_POINT('',(12.16,-5.,1.));
#4930=CARTESIAN_POINT('',(12.16,-5.,-0.1));
#4931=CARTESIAN_POINT('Origin',(12.5,-5.,1.));
#4932=CARTESIAN_POINT('Origin',(12.5,0.,-0.1));
#4933=CARTESIAN_POINT('',(12.16,-4.163799117101E-17,0.));
#4934=CARTESIAN_POINT('Origin',(12.5,0.,0.));
#4935=CARTESIAN_POINT('',(12.16,4.163799117101E-17,1.));
#4936=CARTESIAN_POINT('',(12.16,-4.163799117101E-17,-0.1));
#4937=CARTESIAN_POINT('Origin',(12.5,0.,1.));
#4938=CARTESIAN_POINT('Origin',(12.5,5.,-0.1));
#4939=CARTESIAN_POINT('',(12.16,5.,0.));
#4940=CARTESIAN_POINT('Origin',(12.5,5.,0.));
#4941=CARTESIAN_POINT('',(12.16,5.,1.));
#4942=CARTESIAN_POINT('',(12.16,5.,-0.1));
#4943=CARTESIAN_POINT('Origin',(12.5,5.,1.));
#4944=CARTESIAN_POINT('Origin',(15.,7.5,0.));
#4945=CARTESIAN_POINT('',(15.,7.5,0.));
#4946=CARTESIAN_POINT('',(0.,7.5,0.));
#4947=CARTESIAN_POINT('',(15.,7.5,0.));
#4948=CARTESIAN_POINT('',(0.,7.5,1.));
#4949=CARTESIAN_POINT('',(0.,7.5,0.));
#4950=CARTESIAN_POINT('',(15.,7.5,1.));
#4951=CARTESIAN_POINT('',(15.,7.5,1.));
#4952=CARTESIAN_POINT('',(15.,7.5,0.));
#4953=CARTESIAN_POINT('Origin',(15.,-7.5,0.));
#4954=CARTESIAN_POINT('',(15.,-7.5,0.));
#4955=CARTESIAN_POINT('',(15.,-7.5,0.));
#4956=CARTESIAN_POINT('',(15.,-7.5,1.));
#4957=CARTESIAN_POINT('',(15.,-7.5,1.));
#4958=CARTESIAN_POINT('',(15.,-7.5,0.));
#4959=CARTESIAN_POINT('Origin',(0.,-7.5,0.));
#4960=CARTESIAN_POINT('',(0.,-7.5,0.));
#4961=CARTESIAN_POINT('',(0.,-7.5,0.));
#4962=CARTESIAN_POINT('',(0.,-7.5,1.));
#4963=CARTESIAN_POINT('',(0.,-7.5,1.));
#4964=CARTESIAN_POINT('',(0.,-7.5,0.));
#4965=CARTESIAN_POINT('Origin',(0.,7.5,0.));
#4966=CARTESIAN_POINT('',(0.,7.5,0.));
#4967=CARTESIAN_POINT('',(0.,7.5,1.));
#4968=CARTESIAN_POINT('Origin',(7.5,0.,1.));
#4969=CARTESIAN_POINT('Origin',(7.5,0.,0.));
#5676=UNCERTAINTY_MEASURE_WITH_UNIT(LENGTH_MEASURE(0.001),#5703,
'DISTANCE_ACCURACY_VALUE',
'Maximum model space distance between geometric entities at asserted c
onnectivities');
#5688=UNCERTAINTY_MEASURE_WITH_UNIT(LENGTH_MEASURE(0.001),#5703,
'DISTANCE_ACCURACY_VALUE',
'Maximum model space distance between geometric entities at asserted c
onnectivities');
#5690=(
GEOMETRIC_REPRESENTATION_CONTEXT(3)
GLOBAL_UNCERTAINTY_ASSIGNED_CONTEXT((#5676))
GLOBAL_UNIT_ASSIGNED_CONTEXT((#5703,#5705,#5706))
REPRESENTATION_CONTEXT('','3D')
);
#5702=(
GEOMETRIC_REPRESENTATION_CONTEXT(3)
GLOBAL_UNCERTAINTY_ASSIGNED_CONTEXT((#5688))
GLOBAL_UNIT_ASSIGNED_CONTEXT((#5703,#5705,#5706))
REPRESENTATION_CONTEXT('','3D')
);
#5703=(
LENGTH_UNIT()
NAMED_UNIT(*)
SI_UNIT(.CENTI.,.METRE.)
);
#5705=(
NAMED_UNIT(*)
PLANE_ANGLE_UNIT()
SI_UNIT($,.RADIAN.)
);
#5706=(
NAMED_UNIT(*)
SI_UNIT($,.STERADIAN.)
SOLID_ANGLE_UNIT()
);
#5708=SHAPE_DEFINITION_REPRESENTATION(#5721,#5760);
#5721=PRODUCT_DEFINITION_SHAPE('',$,#5774);
#5760=SHAPE_REPRESENTATION('',(#3411),#5690);
#5772=PRODUCT_DEFINITION_CONTEXT('part definition',#5813,'design');
#5774=PRODUCT_DEFINITION('Fixture grid plate','Fixture grid plate',
#5787,#5772);
#5787=PRODUCT_DEFINITION_FORMATION('',$,#5816);
#5813=APPLICATION_CONTEXT(
'Core Data for Automotive Mechanical Design Process');
#5814=PRODUCT_CONTEXT('part definition',#5813,'mechanical');
#5816=PRODUCT('Fixture grid plate','Fixture grid plate',
'Fixture grid plate',(#5814));
#5905=COLOUR_RGB('Off White',0.89,0.88,0.83);
#5906=FILL_AREA_STYLE_COLOUR('',#5905);
#5907=FILL_AREA_STYLE('',(#5906));
#5908=SURFACE_STYLE_FILL_AREA(#5907);
#5909=SURFACE_SIDE_STYLE('',(#5908));
#5910=SURFACE_STYLE_USAGE(.BOTH.,#5909);
#5911=PRESENTATION_STYLE_ASSIGNMENT((#5910));
ENDSEC;
END-ISO-10303-21;
